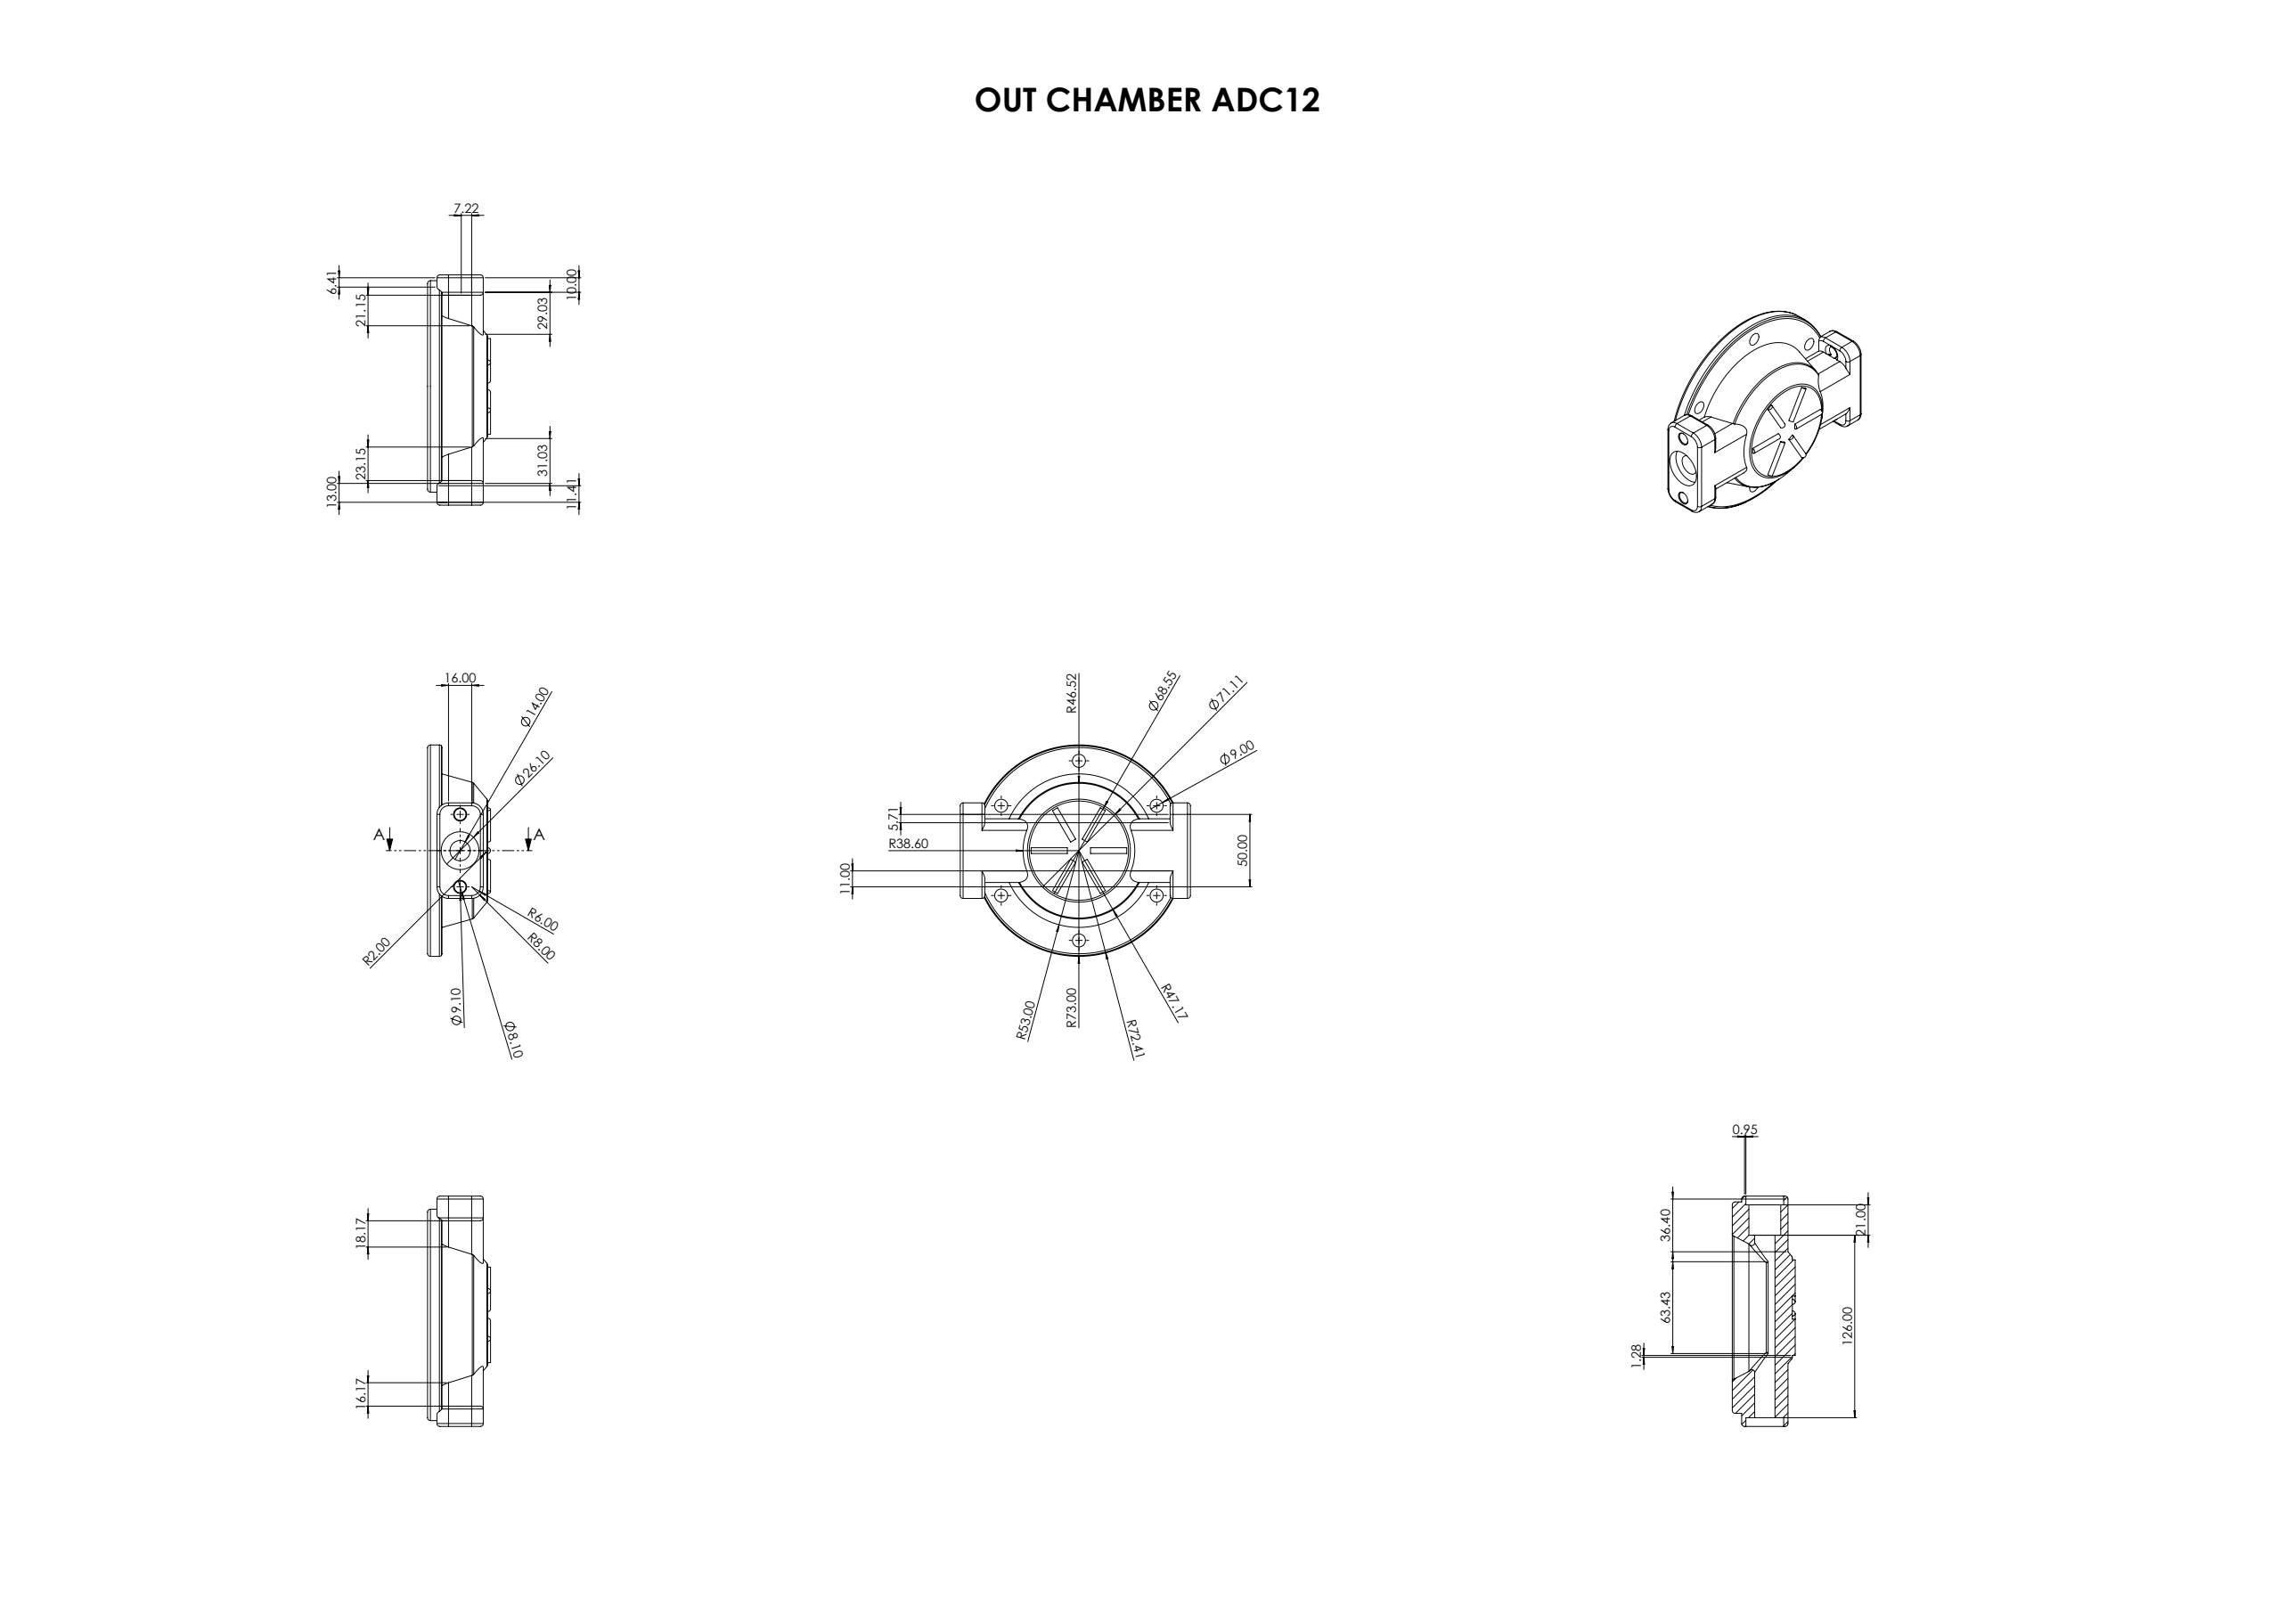
ISO-10303-21;
HEADER;
/* Generated by software containing ST-Developer
 * from STEP Tools, Inc. (www.steptools.com) 
 */

FILE_DESCRIPTION(
/* description */ (''),
/* implementation_level */ '2;1');

FILE_NAME(
/* name */ '01_Out_Chamber_ADC12.step',
/* time_stamp */ '2026-10-26T06:13:19-07:00',
/* author */ (''),
/* organization */ (''),
/* preprocessor_version */ 'ST-DEVELOPER v20.2',
/* originating_system */ 'Autodesk Translation Framework v15.15.0.0',
/* authorisation */ '');

FILE_SCHEMA (('AUTOMOTIVE_DESIGN { 1 0 10303 214 3 1 1 }','TECHNICAL_DATA_PACKAGING'));
ENDSEC;

DATA;
#10=MECHANICAL_DESIGN_GEOMETRIC_PRESENTATION_REPRESENTATION('',(#297),#56639);
#257=SHAPE_REPRESENTATION_RELATIONSHIP('SRR','None',#56745,#277);
#277=ADVANCED_BREP_SHAPE_REPRESENTATION('',(#317),#56619);
#297=STYLED_ITEM('',(#56908),#317);
#317=MANIFOLD_SOLID_BREP('Body1',#16949);
#337=B_SPLINE_SURFACE_WITH_KNOTS('',3,3,((#23722,#23723,#23724,#23725,#23726,
#23727,#23728,#23729,#23730,#23731,#23732,#23733,#23734,#23735),(#23736,
#23737,#23738,#23739,#23740,#23741,#23742,#23743,#23744,#23745,#23746,#23747,
#23748,#23749),(#23750,#23751,#23752,#23753,#23754,#23755,#23756,#23757,
#23758,#23759,#23760,#23761,#23762,#23763),(#23764,#23765,#23766,#23767,
#23768,#23769,#23770,#23771,#23772,#23773,#23774,#23775,#23776,#23777),
(#23778,#23779,#23780,#23781,#23782,#23783,#23784,#23785,#23786,#23787,
#23788,#23789,#23790,#23791),(#23792,#23793,#23794,#23795,#23796,#23797,
#23798,#23799,#23800,#23801,#23802,#23803,#23804,#23805),(#23806,#23807,
#23808,#23809,#23810,#23811,#23812,#23813,#23814,#23815,#23816,#23817,#23818,
#23819)),.UNSPECIFIED.,.F.,.F.,.F.,(4,1,1,1,4),(4,1,1,1,1,1,1,1,1,1,1,4),
(0.,0.285714285714286,0.571428571428571,0.785714285714286,1.),(4.69190485072485,
5.32399487973813,5.95608490875141,6.27212992325805,6.58817493776469,6.79887161410245,
7.00956829044021,7.22026496677797,7.43096164311573,7.85235499579125,8.48444502480452,
9.1165350538178),.UNSPECIFIED.);
#338=B_SPLINE_SURFACE_WITH_KNOTS('',3,3,((#24134,#24135,#24136,#24137,#24138,
#24139,#24140,#24141,#24142,#24143,#24144,#24145,#24146,#24147,#24148),
(#24149,#24150,#24151,#24152,#24153,#24154,#24155,#24156,#24157,#24158,
#24159,#24160,#24161,#24162,#24163),(#24164,#24165,#24166,#24167,#24168,
#24169,#24170,#24171,#24172,#24173,#24174,#24175,#24176,#24177,#24178),
(#24179,#24180,#24181,#24182,#24183,#24184,#24185,#24186,#24187,#24188,
#24189,#24190,#24191,#24192,#24193),(#24194,#24195,#24196,#24197,#24198,
#24199,#24200,#24201,#24202,#24203,#24204,#24205,#24206,#24207,#24208),
(#24209,#24210,#24211,#24212,#24213,#24214,#24215,#24216,#24217,#24218,
#24219,#24220,#24221,#24222,#24223),(#24224,#24225,#24226,#24227,#24228,
#24229,#24230,#24231,#24232,#24233,#24234,#24235,#24236,#24237,#24238)),
 .UNSPECIFIED.,.F.,.F.,.F.,(4,1,1,1,4),(4,1,1,1,1,1,1,1,1,1,1,1,4),(0.,
0.285714285714286,0.571428571428571,0.785714285714286,1.),(4.69190485072485,
5.32399487973813,5.95608490875141,6.27212992325805,6.58817493776469,6.79887161410245,
7.00956829044021,7.22026496677796,7.43096164311572,7.64165831945348,7.85235499579124,
8.48444502480452,9.1165350538178),.UNSPECIFIED.);
#367=TOROIDAL_SURFACE('',#17234,45.2410588351948,2.);
#368=TOROIDAL_SURFACE('',#17239,45.2410588351948,2.);
#369=TOROIDAL_SURFACE('',#17245,34.2759001296373,2.);
#370=TOROIDAL_SURFACE('',#17254,71.1954923578975,2.);
#371=TOROIDAL_SURFACE('',#17261,71.,2.);
#372=TOROIDAL_SURFACE('',#17269,71.1954923578975,2.);
#373=TOROIDAL_SURFACE('',#17276,71.,2.);
#374=TOROIDAL_SURFACE('',#17277,71.,2.);
#375=TOROIDAL_SURFACE('',#17288,6.,2.);
#376=TOROIDAL_SURFACE('',#17294,6.,2.);
#377=TOROIDAL_SURFACE('',#17306,6.00000000000001,2.);
#378=TOROIDAL_SURFACE('',#17311,6.,2.);
#379=TOROIDAL_SURFACE('',#17316,6.,2.);
#380=TOROIDAL_SURFACE('',#17321,6.,2.);
#381=TOROIDAL_SURFACE('',#17333,6.,2.);
#382=TOROIDAL_SURFACE('',#17335,6.00000000000001,2.);
#383=TOROIDAL_SURFACE('',#17340,51.1654934782503,2.);
#384=TOROIDAL_SURFACE('',#17354,6.,2.);
#385=TOROIDAL_SURFACE('',#17360,6.,2.);
#386=TOROIDAL_SURFACE('',#17371,6.05,2.);
#387=TOROIDAL_SURFACE('',#17373,6.00000000000001,2.);
#388=TOROIDAL_SURFACE('',#17379,6.,2.);
#389=TOROIDAL_SURFACE('',#17384,6.,2.);
#390=TOROIDAL_SURFACE('',#17388,6.,2.);
#391=TOROIDAL_SURFACE('',#17398,6.00000000000001,2.);
#392=TOROIDAL_SURFACE('',#17403,6.,2.);
#393=TOROIDAL_SURFACE('',#17412,6.05,2.);
#414=FACE_BOUND('',#2788,.T.);
#415=FACE_BOUND('',#2789,.T.);
#416=FACE_BOUND('',#2790,.T.);
#417=FACE_BOUND('',#2794,.T.);
#418=FACE_BOUND('',#2795,.T.);
#419=FACE_BOUND('',#2796,.T.);
#420=FACE_BOUND('',#2807,.T.);
#421=FACE_BOUND('',#2808,.T.);
#422=FACE_BOUND('',#2809,.T.);
#423=FACE_BOUND('',#2810,.T.);
#424=FACE_BOUND('',#2811,.T.);
#425=FACE_BOUND('',#2812,.T.);
#426=FACE_BOUND('',#2815,.T.);
#427=FACE_BOUND('',#2816,.T.);
#428=FACE_BOUND('',#2817,.T.);
#429=FACE_BOUND('',#2822,.T.);
#430=FACE_BOUND('',#2823,.T.);
#431=FACE_BOUND('',#2824,.T.);
#432=FACE_BOUND('',#2828,.T.);
#433=FACE_BOUND('',#2829,.T.);
#434=FACE_BOUND('',#2830,.T.);
#435=FACE_BOUND('',#2831,.T.);
#436=FACE_BOUND('',#2832,.T.);
#437=FACE_BOUND('',#2833,.T.);
#438=FACE_BOUND('',#2834,.T.);
#439=FACE_BOUND('',#2922,.T.);
#440=FACE_BOUND('',#2925,.T.);
#441=FACE_BOUND('',#2927,.T.);
#564=CONICAL_SURFACE('',#17208,4.3,0.785398163397448);
#565=CONICAL_SURFACE('',#17217,4.3,0.785398163397448);
#566=CONICAL_SURFACE('',#17218,4.3,0.785398163397439);
#567=CONICAL_SURFACE('',#17230,4.3,0.785398163397439);
#568=CONICAL_SURFACE('',#17237,50.,0.272145890531187);
#569=CONICAL_SURFACE('',#17243,50.,0.272145890531187);
#570=CONICAL_SURFACE('',#17250,41.,0.876058050598193);
#571=CONICAL_SURFACE('',#17344,47.,0.477345382373672);
#572=CONICAL_SURFACE('',#17465,38.,0.785398163397448);
#662=CIRCLE('',#17196,4.05);
#663=CIRCLE('',#17197,4.05);
#664=CIRCLE('',#17198,4.05);
#665=CIRCLE('',#17199,4.05);
#666=CIRCLE('',#17204,4.05);
#667=CIRCLE('',#17205,4.05);
#668=CIRCLE('',#17206,4.05);
#669=CIRCLE('',#17207,4.05);
#670=CIRCLE('',#17209,4.55);
#671=CIRCLE('',#17211,6.00000000000001);
#672=CIRCLE('',#17212,6.);
#673=CIRCLE('',#17213,6.);
#674=CIRCLE('',#17214,6.);
#675=CIRCLE('',#17215,4.55);
#676=CIRCLE('',#17216,13.05);
#677=CIRCLE('',#17219,4.55);
#678=CIRCLE('',#17220,4.05);
#679=CIRCLE('',#17222,6.00000000000001);
#680=CIRCLE('',#17223,6.);
#681=CIRCLE('',#17224,6.);
#682=CIRCLE('',#17225,6.);
#683=CIRCLE('',#17226,4.55);
#684=CIRCLE('',#17227,13.05);
#685=CIRCLE('',#17229,4.05);
#686=CIRCLE('',#17231,4.05);
#687=CIRCLE('',#17233,4.05);
#688=CIRCLE('',#17235,47.1674514378614);
#689=CIRCLE('',#17236,46.5214276345237);
#690=CIRCLE('',#17238,53.);
#691=CIRCLE('',#17240,47.1674514378614);
#692=CIRCLE('',#17241,46.5214276345237);
#693=CIRCLE('',#17242,46.5214276345237);
#694=CIRCLE('',#17244,53.);
#695=CIRCLE('',#17246,34.2759001296373);
#696=CIRCLE('',#17247,2.);
#697=CIRCLE('',#17248,35.5562689289663);
#698=CIRCLE('',#17249,35.5562689289663);
#699=CIRCLE('',#17251,38.6);
#700=CIRCLE('',#17252,38.6);
#701=CIRCLE('',#17255,72.4142135623731);
#702=CIRCLE('',#17256,71.1954923578975);
#703=CIRCLE('',#17258,4.5);
#704=CIRCLE('',#17259,4.5);
#705=CIRCLE('',#17260,4.5);
#706=CIRCLE('',#17262,73.);
#707=CIRCLE('',#17263,73.);
#708=CIRCLE('',#17265,73.);
#709=CIRCLE('',#17266,73.);
#710=CIRCLE('',#17267,73.);
#711=CIRCLE('',#17268,73.);
#712=CIRCLE('',#17270,72.4142135623731);
#713=CIRCLE('',#17271,71.1954923578975);
#714=CIRCLE('',#17273,4.5);
#715=CIRCLE('',#17274,4.5);
#716=CIRCLE('',#17275,4.5);
#717=CIRCLE('',#17278,2.);
#718=CIRCLE('',#17279,71.);
#719=CIRCLE('',#17281,4.5);
#720=CIRCLE('',#17282,4.5);
#721=CIRCLE('',#17283,4.5);
#722=CIRCLE('',#17284,4.5);
#723=CIRCLE('',#17285,4.5);
#724=CIRCLE('',#17286,4.5);
#725=CIRCLE('',#17287,51.1654934782503);
#726=CIRCLE('',#17289,6.);
#727=CIRCLE('',#17290,2.);
#728=CIRCLE('',#17291,8.);
#729=CIRCLE('',#17293,2.);
#730=CIRCLE('',#17295,2.);
#731=CIRCLE('',#17296,8.);
#732=CIRCLE('',#17297,6.);
#733=CIRCLE('',#17301,8.);
#734=CIRCLE('',#17302,8.00000000000001);
#735=CIRCLE('',#17304,2.);
#736=CIRCLE('',#17305,2.);
#737=CIRCLE('',#17307,2.);
#738=CIRCLE('',#17308,8.00000000000001);
#739=CIRCLE('',#17310,2.);
#740=CIRCLE('',#17312,2.);
#741=CIRCLE('',#17313,8.);
#742=CIRCLE('',#17315,2.);
#743=CIRCLE('',#17317,2.);
#744=CIRCLE('',#17318,8.);
#745=CIRCLE('',#17320,2.);
#746=CIRCLE('',#17322,8.);
#747=CIRCLE('',#17324,8.);
#748=CIRCLE('',#17327,8.00000000000001);
#749=CIRCLE('',#17329,2.);
#750=CIRCLE('',#17331,2.00000000000001);
#751=CIRCLE('',#17332,2.);
#752=CIRCLE('',#17334,6.);
#753=CIRCLE('',#17336,6.00000000000001);
#754=CIRCLE('',#17338,8.00000000000002);
#755=CIRCLE('',#17339,8.00000000000001);
#756=CIRCLE('',#17341,2.);
#757=CIRCLE('',#17342,49.3890581919384);
#758=CIRCLE('',#17343,49.3890581919384);
#759=CIRCLE('',#17345,44.);
#760=CIRCLE('',#17349,32.);
#761=CIRCLE('',#17350,32.);
#762=CIRCLE('',#17352,7.);
#763=CIRCLE('',#17353,7.);
#764=CIRCLE('',#17355,8.);
#765=CIRCLE('',#17356,2.);
#766=CIRCLE('',#17357,6.);
#767=CIRCLE('',#17359,2.);
#768=CIRCLE('',#17361,1.99999999999999);
#769=CIRCLE('',#17362,6.);
#770=CIRCLE('',#17363,8.);
#771=CIRCLE('',#17367,8.);
#772=CIRCLE('',#17369,6.05);
#773=CIRCLE('',#17370,8.);
#774=CIRCLE('',#17372,6.05);
#775=CIRCLE('',#17374,2.);
#776=CIRCLE('',#17375,2.);
#777=CIRCLE('',#17376,8.00000000000001);
#778=CIRCLE('',#17378,2.);
#779=CIRCLE('',#17380,2.);
#780=CIRCLE('',#17381,8.);
#781=CIRCLE('',#17383,2.);
#782=CIRCLE('',#17385,2.);
#783=CIRCLE('',#17387,2.);
#784=CIRCLE('',#17389,2.);
#785=CIRCLE('',#17390,8.);
#786=CIRCLE('',#17395,8.00000000000001);
#787=CIRCLE('',#17397,2.);
#788=CIRCLE('',#17399,2.);
#789=CIRCLE('',#17400,6.00000000000001);
#790=CIRCLE('',#17402,2.);
#791=CIRCLE('',#17404,6.);
#792=CIRCLE('',#17405,8.);
#793=CIRCLE('',#17407,8.00000000000001);
#794=CIRCLE('',#17408,6.05);
#795=CIRCLE('',#17410,6.05);
#796=CIRCLE('',#17411,8.00000000000002);
#797=CIRCLE('',#17414,2.);
#798=CIRCLE('',#17416,2.);
#799=CIRCLE('',#17418,2.);
#800=CIRCLE('',#17420,2.);
#801=CIRCLE('',#17422,2.);
#802=CIRCLE('',#17424,2.);
#803=CIRCLE('',#17426,2.);
#804=CIRCLE('',#17428,2.);
#805=CIRCLE('',#17430,2.);
#806=CIRCLE('',#17432,2.);
#807=CIRCLE('',#17434,2.);
#808=CIRCLE('',#17436,2.);
#809=CIRCLE('',#17448,8.00000000000001);
#810=CIRCLE('',#17456,13.05);
#811=CIRCLE('',#17458,11.);
#812=CIRCLE('',#17460,11.);
#813=CIRCLE('',#17463,13.05);
#814=CIRCLE('',#17466,32.);
#1226=CYLINDRICAL_SURFACE('',#17195,4.05);
#1227=CYLINDRICAL_SURFACE('',#17203,4.05);
#1228=CYLINDRICAL_SURFACE('',#17228,4.05);
#1229=CYLINDRICAL_SURFACE('',#17232,4.05);
#1230=CYLINDRICAL_SURFACE('',#17264,73.);
#1231=CYLINDRICAL_SURFACE('',#17292,2.);
#1232=CYLINDRICAL_SURFACE('',#17298,2.);
#1233=CYLINDRICAL_SURFACE('',#17303,2.);
#1234=CYLINDRICAL_SURFACE('',#17309,2.);
#1235=CYLINDRICAL_SURFACE('',#17314,2.);
#1236=CYLINDRICAL_SURFACE('',#17319,2.);
#1237=CYLINDRICAL_SURFACE('',#17323,8.);
#1238=CYLINDRICAL_SURFACE('',#17326,8.00000000000001);
#1239=CYLINDRICAL_SURFACE('',#17328,2.);
#1240=CYLINDRICAL_SURFACE('',#17330,2.);
#1241=CYLINDRICAL_SURFACE('',#17346,2.);
#1242=CYLINDRICAL_SURFACE('',#17347,2.);
#1243=CYLINDRICAL_SURFACE('',#17351,7.);
#1244=CYLINDRICAL_SURFACE('',#17358,2.);
#1245=CYLINDRICAL_SURFACE('',#17364,2.);
#1246=CYLINDRICAL_SURFACE('',#17366,8.);
#1247=CYLINDRICAL_SURFACE('',#17377,2.);
#1248=CYLINDRICAL_SURFACE('',#17382,2.);
#1249=CYLINDRICAL_SURFACE('',#17386,2.);
#1250=CYLINDRICAL_SURFACE('',#17391,2.);
#1251=CYLINDRICAL_SURFACE('',#17392,8.);
#1252=CYLINDRICAL_SURFACE('',#17394,8.00000000000001);
#1253=CYLINDRICAL_SURFACE('',#17396,2.);
#1254=CYLINDRICAL_SURFACE('',#17401,2.);
#1255=CYLINDRICAL_SURFACE('',#17415,2.);
#1256=CYLINDRICAL_SURFACE('',#17419,2.);
#1257=CYLINDRICAL_SURFACE('',#17423,2.);
#1258=CYLINDRICAL_SURFACE('',#17427,2.);
#1259=CYLINDRICAL_SURFACE('',#17431,2.);
#1260=CYLINDRICAL_SURFACE('',#17435,2.);
#1261=CYLINDRICAL_SURFACE('',#17449,4.5);
#1262=CYLINDRICAL_SURFACE('',#17450,4.5);
#1263=CYLINDRICAL_SURFACE('',#17451,4.5);
#1264=CYLINDRICAL_SURFACE('',#17452,4.5);
#1265=CYLINDRICAL_SURFACE('',#17453,4.5);
#1266=CYLINDRICAL_SURFACE('',#17454,4.5);
#1267=CYLINDRICAL_SURFACE('',#17455,13.05);
#1268=CYLINDRICAL_SURFACE('',#17459,11.);
#1269=CYLINDRICAL_SURFACE('',#17464,13.05);
#1270=CYLINDRICAL_SURFACE('',#17468,8.);
#1271=CYLINDRICAL_SURFACE('',#17470,8.);
#1272=CYLINDRICAL_SURFACE('',#17471,8.);
#1273=CYLINDRICAL_SURFACE('',#17473,8.00000000000001);
#1274=CYLINDRICAL_SURFACE('',#17476,8.);
#1275=CYLINDRICAL_SURFACE('',#17477,8.);
#1276=CYLINDRICAL_SURFACE('',#17478,8.00000000000002);
#1277=CYLINDRICAL_SURFACE('',#17479,8.00000000000001);
#1278=CYLINDRICAL_SURFACE('',#17481,8.00000000000001);
#1279=CYLINDRICAL_SURFACE('',#17483,8.00000000000002);
#1280=CYLINDRICAL_SURFACE('',#17484,8.00000000000001);
#1761=(
BOUNDED_CURVE()
B_SPLINE_CURVE(2,(#22976,#22977,#22978),.UNSPECIFIED.,.F.,.F.)
B_SPLINE_CURVE_WITH_KNOTS((3,3),(0.,1.67588266328234),.UNSPECIFIED.)
CURVE()
GEOMETRIC_REPRESENTATION_ITEM()
RATIONAL_B_SPLINE_CURVE((1.,1.00126993326289,1.))
REPRESENTATION_ITEM('')
);
#1762=(
BOUNDED_CURVE()
B_SPLINE_CURVE(2,(#23047,#23048,#23049),.UNSPECIFIED.,.F.,.F.)
B_SPLINE_CURVE_WITH_KNOTS((3,3),(0.,1.67588266328234),.UNSPECIFIED.)
CURVE()
GEOMETRIC_REPRESENTATION_ITEM()
RATIONAL_B_SPLINE_CURVE((1.,1.00126993326289,1.))
REPRESENTATION_ITEM('')
);
#1763=(
BOUNDED_CURVE()
B_SPLINE_CURVE(2,(#23196,#23197,#23198),.UNSPECIFIED.,.F.,.F.)
B_SPLINE_CURVE_WITH_KNOTS((3,3),(0.,1.67588266328234),.UNSPECIFIED.)
CURVE()
GEOMETRIC_REPRESENTATION_ITEM()
RATIONAL_B_SPLINE_CURVE((1.,1.00126993326289,1.))
REPRESENTATION_ITEM('')
);
#1764=(
BOUNDED_CURVE()
B_SPLINE_CURVE(2,(#23235,#23236,#23237),.UNSPECIFIED.,.F.,.F.)
B_SPLINE_CURVE_WITH_KNOTS((3,3),(0.,1.67588266328234),.UNSPECIFIED.)
CURVE()
GEOMETRIC_REPRESENTATION_ITEM()
RATIONAL_B_SPLINE_CURVE((1.,1.00126993326289,1.))
REPRESENTATION_ITEM('')
);
#1805=FACE_OUTER_BOUND('',#2778,.T.);
#1806=FACE_OUTER_BOUND('',#2779,.T.);
#1807=FACE_OUTER_BOUND('',#2780,.T.);
#1808=FACE_OUTER_BOUND('',#2781,.T.);
#1809=FACE_OUTER_BOUND('',#2782,.T.);
#1810=FACE_OUTER_BOUND('',#2783,.T.);
#1811=FACE_OUTER_BOUND('',#2784,.T.);
#1812=FACE_OUTER_BOUND('',#2785,.T.);
#1813=FACE_OUTER_BOUND('',#2786,.T.);
#1814=FACE_OUTER_BOUND('',#2787,.T.);
#1815=FACE_OUTER_BOUND('',#2791,.T.);
#1816=FACE_OUTER_BOUND('',#2792,.T.);
#1817=FACE_OUTER_BOUND('',#2793,.T.);
#1818=FACE_OUTER_BOUND('',#2797,.T.);
#1819=FACE_OUTER_BOUND('',#2798,.T.);
#1820=FACE_OUTER_BOUND('',#2799,.T.);
#1821=FACE_OUTER_BOUND('',#2800,.T.);
#1822=FACE_OUTER_BOUND('',#2801,.T.);
#1823=FACE_OUTER_BOUND('',#2802,.T.);
#1824=FACE_OUTER_BOUND('',#2803,.T.);
#1825=FACE_OUTER_BOUND('',#2804,.T.);
#1826=FACE_OUTER_BOUND('',#2805,.T.);
#1827=FACE_OUTER_BOUND('',#2806,.T.);
#1828=FACE_OUTER_BOUND('',#2813,.T.);
#1829=FACE_OUTER_BOUND('',#2814,.T.);
#1830=FACE_OUTER_BOUND('',#2818,.T.);
#1831=FACE_OUTER_BOUND('',#2819,.T.);
#1832=FACE_OUTER_BOUND('',#2820,.T.);
#1833=FACE_OUTER_BOUND('',#2821,.T.);
#1834=FACE_OUTER_BOUND('',#2825,.T.);
#1835=FACE_OUTER_BOUND('',#2826,.T.);
#1836=FACE_OUTER_BOUND('',#2827,.T.);
#1837=FACE_OUTER_BOUND('',#2835,.T.);
#1838=FACE_OUTER_BOUND('',#2836,.T.);
#1839=FACE_OUTER_BOUND('',#2837,.T.);
#1840=FACE_OUTER_BOUND('',#2838,.T.);
#1841=FACE_OUTER_BOUND('',#2839,.T.);
#1842=FACE_OUTER_BOUND('',#2840,.T.);
#1843=FACE_OUTER_BOUND('',#2841,.T.);
#1844=FACE_OUTER_BOUND('',#2842,.T.);
#1845=FACE_OUTER_BOUND('',#2843,.T.);
#1846=FACE_OUTER_BOUND('',#2844,.T.);
#1847=FACE_OUTER_BOUND('',#2845,.T.);
#1848=FACE_OUTER_BOUND('',#2846,.T.);
#1849=FACE_OUTER_BOUND('',#2847,.T.);
#1850=FACE_OUTER_BOUND('',#2848,.T.);
#1851=FACE_OUTER_BOUND('',#2849,.T.);
#1852=FACE_OUTER_BOUND('',#2850,.T.);
#1853=FACE_OUTER_BOUND('',#2851,.T.);
#1854=FACE_OUTER_BOUND('',#2852,.T.);
#1855=FACE_OUTER_BOUND('',#2853,.T.);
#1856=FACE_OUTER_BOUND('',#2854,.T.);
#1857=FACE_OUTER_BOUND('',#2855,.T.);
#1858=FACE_OUTER_BOUND('',#2856,.T.);
#1859=FACE_OUTER_BOUND('',#2857,.T.);
#1860=FACE_OUTER_BOUND('',#2858,.T.);
#1861=FACE_OUTER_BOUND('',#2859,.T.);
#1862=FACE_OUTER_BOUND('',#2860,.T.);
#1863=FACE_OUTER_BOUND('',#2861,.T.);
#1864=FACE_OUTER_BOUND('',#2862,.T.);
#1865=FACE_OUTER_BOUND('',#2863,.T.);
#1866=FACE_OUTER_BOUND('',#2864,.T.);
#1867=FACE_OUTER_BOUND('',#2865,.T.);
#1868=FACE_OUTER_BOUND('',#2866,.T.);
#1869=FACE_OUTER_BOUND('',#2867,.T.);
#1870=FACE_OUTER_BOUND('',#2868,.T.);
#1871=FACE_OUTER_BOUND('',#2869,.T.);
#1872=FACE_OUTER_BOUND('',#2870,.T.);
#1873=FACE_OUTER_BOUND('',#2871,.T.);
#1874=FACE_OUTER_BOUND('',#2872,.T.);
#1875=FACE_OUTER_BOUND('',#2873,.T.);
#1876=FACE_OUTER_BOUND('',#2874,.T.);
#1877=FACE_OUTER_BOUND('',#2875,.T.);
#1878=FACE_OUTER_BOUND('',#2876,.T.);
#1879=FACE_OUTER_BOUND('',#2877,.T.);
#1880=FACE_OUTER_BOUND('',#2878,.T.);
#1881=FACE_OUTER_BOUND('',#2879,.T.);
#1882=FACE_OUTER_BOUND('',#2880,.T.);
#1883=FACE_OUTER_BOUND('',#2881,.T.);
#1884=FACE_OUTER_BOUND('',#2882,.T.);
#1885=FACE_OUTER_BOUND('',#2883,.T.);
#1886=FACE_OUTER_BOUND('',#2884,.T.);
#1887=FACE_OUTER_BOUND('',#2885,.T.);
#1888=FACE_OUTER_BOUND('',#2886,.T.);
#1889=FACE_OUTER_BOUND('',#2887,.T.);
#1890=FACE_OUTER_BOUND('',#2888,.T.);
#1891=FACE_OUTER_BOUND('',#2889,.T.);
#1892=FACE_OUTER_BOUND('',#2890,.T.);
#1893=FACE_OUTER_BOUND('',#2891,.T.);
#1894=FACE_OUTER_BOUND('',#2892,.T.);
#1895=FACE_OUTER_BOUND('',#2893,.T.);
#1896=FACE_OUTER_BOUND('',#2894,.T.);
#1897=FACE_OUTER_BOUND('',#2895,.T.);
#1898=FACE_OUTER_BOUND('',#2896,.T.);
#1899=FACE_OUTER_BOUND('',#2897,.T.);
#1900=FACE_OUTER_BOUND('',#2898,.T.);
#1901=FACE_OUTER_BOUND('',#2899,.T.);
#1902=FACE_OUTER_BOUND('',#2900,.T.);
#1903=FACE_OUTER_BOUND('',#2901,.T.);
#1904=FACE_OUTER_BOUND('',#2902,.T.);
#1905=FACE_OUTER_BOUND('',#2903,.T.);
#1906=FACE_OUTER_BOUND('',#2904,.T.);
#1907=FACE_OUTER_BOUND('',#2905,.T.);
#1908=FACE_OUTER_BOUND('',#2906,.T.);
#1909=FACE_OUTER_BOUND('',#2907,.T.);
#1910=FACE_OUTER_BOUND('',#2908,.T.);
#1911=FACE_OUTER_BOUND('',#2909,.T.);
#1912=FACE_OUTER_BOUND('',#2910,.T.);
#1913=FACE_OUTER_BOUND('',#2911,.T.);
#1914=FACE_OUTER_BOUND('',#2912,.T.);
#1915=FACE_OUTER_BOUND('',#2913,.T.);
#1916=FACE_OUTER_BOUND('',#2914,.T.);
#1917=FACE_OUTER_BOUND('',#2915,.T.);
#1918=FACE_OUTER_BOUND('',#2916,.T.);
#1919=FACE_OUTER_BOUND('',#2917,.T.);
#1920=FACE_OUTER_BOUND('',#2918,.T.);
#1921=FACE_OUTER_BOUND('',#2919,.T.);
#1922=FACE_OUTER_BOUND('',#2920,.T.);
#1923=FACE_OUTER_BOUND('',#2921,.T.);
#1924=FACE_OUTER_BOUND('',#2923,.T.);
#1925=FACE_OUTER_BOUND('',#2924,.T.);
#1926=FACE_OUTER_BOUND('',#2926,.T.);
#1927=FACE_OUTER_BOUND('',#2928,.T.);
#1928=FACE_OUTER_BOUND('',#2929,.T.);
#1929=FACE_OUTER_BOUND('',#2930,.T.);
#1930=FACE_OUTER_BOUND('',#2931,.T.);
#1931=FACE_OUTER_BOUND('',#2932,.T.);
#1932=FACE_OUTER_BOUND('',#2933,.T.);
#1933=FACE_OUTER_BOUND('',#2934,.T.);
#1934=FACE_OUTER_BOUND('',#2935,.T.);
#1935=FACE_OUTER_BOUND('',#2936,.T.);
#1936=FACE_OUTER_BOUND('',#2937,.T.);
#1937=FACE_OUTER_BOUND('',#2938,.T.);
#1938=FACE_OUTER_BOUND('',#2939,.T.);
#1939=FACE_OUTER_BOUND('',#2940,.T.);
#1940=FACE_OUTER_BOUND('',#2941,.T.);
#1941=FACE_OUTER_BOUND('',#2942,.T.);
#1942=FACE_OUTER_BOUND('',#2943,.T.);
#1943=FACE_OUTER_BOUND('',#2944,.T.);
#1944=FACE_OUTER_BOUND('',#2945,.T.);
#1945=FACE_OUTER_BOUND('',#2946,.T.);
#1946=FACE_OUTER_BOUND('',#2947,.T.);
#2778=EDGE_LOOP('',(#10764,#10765,#10766,#10767));
#2779=EDGE_LOOP('',(#10768,#10769,#10770,#10771,#10772,#10773,#10774,#10775,
#10776,#10777));
#2780=EDGE_LOOP('',(#10778,#10779,#10780,#10781));
#2781=EDGE_LOOP('',(#10782,#10783,#10784,#10785,#10786,#10787,#10788,#10789));
#2782=EDGE_LOOP('',(#10790,#10791,#10792,#10793));
#2783=EDGE_LOOP('',(#10794,#10795,#10796,#10797,#10798,#10799,#10800,#10801,
#10802,#10803));
#2784=EDGE_LOOP('',(#10804,#10805,#10806,#10807));
#2785=EDGE_LOOP('',(#10808,#10809,#10810,#10811,#10812,#10813,#10814,#10815));
#2786=EDGE_LOOP('',(#10816,#10817,#10818,#10819));
#2787=EDGE_LOOP('',(#10820,#10821,#10822,#10823,#10824,#10825,#10826,#10827));
#2788=EDGE_LOOP('',(#10828));
#2789=EDGE_LOOP('',(#10829));
#2790=EDGE_LOOP('',(#10830));
#2791=EDGE_LOOP('',(#10831,#10832,#10833,#10834));
#2792=EDGE_LOOP('',(#10835,#10836,#10837,#10838));
#2793=EDGE_LOOP('',(#10839,#10840,#10841,#10842,#10843,#10844,#10845,#10846));
#2794=EDGE_LOOP('',(#10847));
#2795=EDGE_LOOP('',(#10848));
#2796=EDGE_LOOP('',(#10849));
#2797=EDGE_LOOP('',(#10850,#10851,#10852,#10853));
#2798=EDGE_LOOP('',(#10854,#10855,#10856,#10857));
#2799=EDGE_LOOP('',(#10858,#10859,#10860,#10861));
#2800=EDGE_LOOP('',(#10862,#10863,#10864,#10865));
#2801=EDGE_LOOP('',(#10866,#10867,#10868,#10869,#10870,#10871,#10872,#10873));
#2802=EDGE_LOOP('',(#10874,#10875,#10876,#10877,#10878));
#2803=EDGE_LOOP('',(#10879,#10880,#10881,#10882,#10883,#10884,#10885,#10886));
#2804=EDGE_LOOP('',(#10887,#10888,#10889,#10890,#10891));
#2805=EDGE_LOOP('',(#10892,#10893,#10894,#10895,#10896,#10897,#10898,#10899,
#10900,#10901,#10902,#10903,#10904));
#2806=EDGE_LOOP('',(#10905));
#2807=EDGE_LOOP('',(#10906,#10907,#10908,#10909));
#2808=EDGE_LOOP('',(#10910,#10911,#10912,#10913));
#2809=EDGE_LOOP('',(#10914,#10915,#10916,#10917));
#2810=EDGE_LOOP('',(#10918,#10919,#10920,#10921));
#2811=EDGE_LOOP('',(#10922,#10923,#10924,#10925));
#2812=EDGE_LOOP('',(#10926,#10927,#10928,#10929));
#2813=EDGE_LOOP('',(#10930,#10931,#10932,#10933,#10934));
#2814=EDGE_LOOP('',(#10935,#10936,#10937,#10938,#10939,#10940,#10941,#10942));
#2815=EDGE_LOOP('',(#10943));
#2816=EDGE_LOOP('',(#10944));
#2817=EDGE_LOOP('',(#10945));
#2818=EDGE_LOOP('',(#10946,#10947,#10948,#10949,#10950));
#2819=EDGE_LOOP('',(#10951,#10952,#10953,#10954,#10955,#10956,#10957,#10958,
#10959,#10960,#10961,#10962,#10963,#10964));
#2820=EDGE_LOOP('',(#10965,#10966,#10967,#10968,#10969));
#2821=EDGE_LOOP('',(#10970,#10971,#10972,#10973,#10974,#10975,#10976,#10977));
#2822=EDGE_LOOP('',(#10978));
#2823=EDGE_LOOP('',(#10979));
#2824=EDGE_LOOP('',(#10980));
#2825=EDGE_LOOP('',(#10981,#10982,#10983,#10984));
#2826=EDGE_LOOP('',(#10985,#10986,#10987,#10988));
#2827=EDGE_LOOP('',(#10989));
#2828=EDGE_LOOP('',(#10990));
#2829=EDGE_LOOP('',(#10991));
#2830=EDGE_LOOP('',(#10992));
#2831=EDGE_LOOP('',(#10993));
#2832=EDGE_LOOP('',(#10994));
#2833=EDGE_LOOP('',(#10995));
#2834=EDGE_LOOP('',(#10996));
#2835=EDGE_LOOP('',(#10997,#10998,#10999,#11000,#11001,#11002,#11003));
#2836=EDGE_LOOP('',(#11004,#11005,#11006,#11007));
#2837=EDGE_LOOP('',(#11008,#11009,#11010,#11011));
#2838=EDGE_LOOP('',(#11012,#11013,#11014,#11015));
#2839=EDGE_LOOP('',(#11016,#11017,#11018,#11019,#11020,#11021,#11022,#11023));
#2840=EDGE_LOOP('',(#11024,#11025,#11026,#11027,#11028,#11029,#11030,#11031));
#2841=EDGE_LOOP('',(#11032,#11033,#11034,#11035));
#2842=EDGE_LOOP('',(#11036,#11037,#11038,#11039));
#2843=EDGE_LOOP('',(#11040,#11041,#11042,#11043));
#2844=EDGE_LOOP('',(#11044,#11045,#11046,#11047));
#2845=EDGE_LOOP('',(#11048,#11049,#11050,#11051));
#2846=EDGE_LOOP('',(#11052,#11053,#11054,#11055));
#2847=EDGE_LOOP('',(#11056,#11057,#11058,#11059));
#2848=EDGE_LOOP('',(#11060,#11061,#11062,#11063));
#2849=EDGE_LOOP('',(#11064,#11065,#11066,#11067,#11068));
#2850=EDGE_LOOP('',(#11069,#11070,#11071,#11072));
#2851=EDGE_LOOP('',(#11073,#11074,#11075,#11076));
#2852=EDGE_LOOP('',(#11077,#11078,#11079,#11080));
#2853=EDGE_LOOP('',(#11081,#11082,#11083,#11084));
#2854=EDGE_LOOP('',(#11085,#11086,#11087,#11088,#11089,#11090,#11091));
#2855=EDGE_LOOP('',(#11092,#11093,#11094,#11095));
#2856=EDGE_LOOP('',(#11096,#11097,#11098,#11099,#11100,#11101,#11102,#11103));
#2857=EDGE_LOOP('',(#11104,#11105,#11106,#11107,#11108));
#2858=EDGE_LOOP('',(#11109,#11110,#11111,#11112,#11113));
#2859=EDGE_LOOP('',(#11114,#11115,#11116,#11117,#11118,#11119,#11120));
#2860=EDGE_LOOP('',(#11121,#11122,#11123,#11124,#11125,#11126));
#2861=EDGE_LOOP('',(#11127,#11128,#11129,#11130,#11131,#11132));
#2862=EDGE_LOOP('',(#11133,#11134,#11135,#11136,#11137,#11138,#11139));
#2863=EDGE_LOOP('',(#11140,#11141,#11142));
#2864=EDGE_LOOP('',(#11143,#11144,#11145,#11146,#11147,#11148,#11149,#11150,
#11151,#11152,#11153,#11154));
#2865=EDGE_LOOP('',(#11155,#11156,#11157,#11158,#11159));
#2866=EDGE_LOOP('',(#11160,#11161,#11162,#11163,#11164,#11165));
#2867=EDGE_LOOP('',(#11166,#11167,#11168,#11169));
#2868=EDGE_LOOP('',(#11170,#11171,#11172,#11173));
#2869=EDGE_LOOP('',(#11174,#11175,#11176,#11177));
#2870=EDGE_LOOP('',(#11178,#11179,#11180,#11181,#11182,#11183,#11184));
#2871=EDGE_LOOP('',(#11185,#11186,#11187,#11188,#11189,#11190));
#2872=EDGE_LOOP('',(#11191,#11192,#11193,#11194,#11195,#11196,#11197,#11198,
#11199));
#2873=EDGE_LOOP('',(#11200,#11201,#11202,#11203));
#2874=EDGE_LOOP('',(#11204,#11205,#11206,#11207));
#2875=EDGE_LOOP('',(#11208,#11209,#11210,#11211));
#2876=EDGE_LOOP('',(#11212,#11213,#11214,#11215));
#2877=EDGE_LOOP('',(#11216,#11217,#11218,#11219));
#2878=EDGE_LOOP('',(#11220,#11221,#11222,#11223));
#2879=EDGE_LOOP('',(#11224,#11225,#11226,#11227));
#2880=EDGE_LOOP('',(#11228,#11229,#11230,#11231));
#2881=EDGE_LOOP('',(#11232,#11233,#11234,#11235));
#2882=EDGE_LOOP('',(#11236,#11237,#11238,#11239,#11240,#11241,#11242,#11243));
#2883=EDGE_LOOP('',(#11244,#11245,#11246,#11247));
#2884=EDGE_LOOP('',(#11248,#11249,#11250,#11251));
#2885=EDGE_LOOP('',(#11252,#11253,#11254,#11255));
#2886=EDGE_LOOP('',(#11256,#11257,#11258,#11259,#11260,#11261));
#2887=EDGE_LOOP('',(#11262,#11263,#11264,#11265,#11266));
#2888=EDGE_LOOP('',(#11267,#11268,#11269,#11270,#11271,#11272));
#2889=EDGE_LOOP('',(#11273,#11274,#11275,#11276,#11277,#11278));
#2890=EDGE_LOOP('',(#11279,#11280,#11281,#11282,#11283,#11284,#11285,#11286,
#11287));
#2891=EDGE_LOOP('',(#11288,#11289));
#2892=EDGE_LOOP('',(#11290,#11291,#11292,#11293));
#2893=EDGE_LOOP('',(#11294,#11295));
#2894=EDGE_LOOP('',(#11296,#11297,#11298,#11299));
#2895=EDGE_LOOP('',(#11300,#11301));
#2896=EDGE_LOOP('',(#11302,#11303,#11304,#11305));
#2897=EDGE_LOOP('',(#11306,#11307));
#2898=EDGE_LOOP('',(#11308,#11309,#11310,#11311));
#2899=EDGE_LOOP('',(#11312,#11313));
#2900=EDGE_LOOP('',(#11314,#11315,#11316,#11317));
#2901=EDGE_LOOP('',(#11318,#11319));
#2902=EDGE_LOOP('',(#11320,#11321,#11322,#11323));
#2903=EDGE_LOOP('',(#11324,#11325));
#2904=EDGE_LOOP('',(#11326,#11327));
#2905=EDGE_LOOP('',(#11328,#11329));
#2906=EDGE_LOOP('',(#11330,#11331));
#2907=EDGE_LOOP('',(#11332,#11333));
#2908=EDGE_LOOP('',(#11334,#11335));
#2909=EDGE_LOOP('',(#11336));
#2910=EDGE_LOOP('',(#11337));
#2911=EDGE_LOOP('',(#11338,#11339,#11340,#11341));
#2912=EDGE_LOOP('',(#11342,#11343,#11344,#11345));
#2913=EDGE_LOOP('',(#11346,#11347,#11348,#11349,#11350,#11351));
#2914=EDGE_LOOP('',(#11352,#11353,#11354,#11355));
#2915=EDGE_LOOP('',(#11356,#11357,#11358,#11359));
#2916=EDGE_LOOP('',(#11360,#11361,#11362,#11363));
#2917=EDGE_LOOP('',(#11364,#11365,#11366,#11367));
#2918=EDGE_LOOP('',(#11368,#11369,#11370,#11371));
#2919=EDGE_LOOP('',(#11372,#11373,#11374,#11375));
#2920=EDGE_LOOP('',(#11376,#11377,#11378,#11379));
#2921=EDGE_LOOP('',(#11380));
#2922=EDGE_LOOP('',(#11381));
#2923=EDGE_LOOP('',(#11382,#11383,#11384,#11385));
#2924=EDGE_LOOP('',(#11386));
#2925=EDGE_LOOP('',(#11387));
#2926=EDGE_LOOP('',(#11388));
#2927=EDGE_LOOP('',(#11389));
#2928=EDGE_LOOP('',(#11390,#11391,#11392,#11393));
#2929=EDGE_LOOP('',(#11394,#11395,#11396,#11397,#11398,#11399,#11400,#11401,
#11402,#11403,#11404,#11405,#11406,#11407,#11408,#11409));
#2930=EDGE_LOOP('',(#11410,#11411));
#2931=EDGE_LOOP('',(#11412,#11413,#11414,#11415));
#2932=EDGE_LOOP('',(#11416,#11417,#11418,#11419));
#2933=EDGE_LOOP('',(#11420,#11421,#11422,#11423,#11424));
#2934=EDGE_LOOP('',(#11425,#11426,#11427,#11428,#11429,#11430,#11431));
#2935=EDGE_LOOP('',(#11432,#11433,#11434,#11435));
#2936=EDGE_LOOP('',(#11436,#11437,#11438,#11439));
#2937=EDGE_LOOP('',(#11440,#11441,#11442,#11443));
#2938=EDGE_LOOP('',(#11444,#11445,#11446,#11447));
#2939=EDGE_LOOP('',(#11448,#11449,#11450,#11451));
#2940=EDGE_LOOP('',(#11452,#11453,#11454,#11455));
#2941=EDGE_LOOP('',(#11456,#11457,#11458,#11459,#11460,#11461,#11462));
#2942=EDGE_LOOP('',(#11463,#11464,#11465,#11466,#11467,#11468,#11469));
#2943=EDGE_LOOP('',(#11470,#11471,#11472,#11473));
#2944=EDGE_LOOP('',(#11474,#11475,#11476,#11477));
#2945=EDGE_LOOP('',(#11478,#11479,#11480,#11481));
#2946=EDGE_LOOP('',(#11482,#11483,#11484,#11485,#11486,#11487,#11488));
#2947=EDGE_LOOP('',(#11489,#11490,#11491,#11492,#11493,#11494,#11495));
#3901=LINE('',#22955,#4855);
#3902=LINE('',#22957,#4856);
#3903=LINE('',#22958,#4857);
#3904=LINE('',#22961,#4858);
#3905=LINE('',#22972,#4859);
#3906=LINE('',#22974,#4860);
#3907=LINE('',#22980,#4861);
#3908=LINE('',#22982,#4862);
#3909=LINE('',#22992,#4863);
#3910=LINE('',#23004,#4864);
#3911=LINE('',#23005,#4865);
#3912=LINE('',#23010,#4866);
#3913=LINE('',#23026,#4867);
#3914=LINE('',#23028,#4868);
#3915=LINE('',#23029,#4869);
#3916=LINE('',#23032,#4870);
#3917=LINE('',#23043,#4871);
#3918=LINE('',#23045,#4872);
#3919=LINE('',#23051,#4873);
#3920=LINE('',#23053,#4874);
#3921=LINE('',#23063,#4875);
#3922=LINE('',#23075,#4876);
#3923=LINE('',#23076,#4877);
#3924=LINE('',#23081,#4878);
#3925=LINE('',#23088,#4879);
#3926=LINE('',#23094,#4880);
#3927=LINE('',#23098,#4881);
#3928=LINE('',#23102,#4882);
#3929=LINE('',#23105,#4883);
#3930=LINE('',#23111,#4884);
#3931=LINE('',#23116,#4885);
#3932=LINE('',#23121,#4886);
#3933=LINE('',#23125,#4887);
#3934=LINE('',#23129,#4888);
#3935=LINE('',#23133,#4889);
#3936=LINE('',#23141,#4890);
#3937=LINE('',#23145,#4891);
#3938=LINE('',#23149,#4892);
#3939=LINE('',#23266,#4893);
#3940=LINE('',#23334,#4894);
#3941=LINE('',#23336,#4895);
#3942=LINE('',#23338,#4896);
#3943=LINE('',#23339,#4897);
#3944=LINE('',#23342,#4898);
#3945=LINE('',#23344,#4899);
#3946=LINE('',#23346,#4900);
#3947=LINE('',#23347,#4901);
#3948=LINE('',#23350,#4902);
#3949=LINE('',#23352,#4903);
#3950=LINE('',#23354,#4904);
#3951=LINE('',#23355,#4905);
#3952=LINE('',#23358,#4906);
#3953=LINE('',#23360,#4907);
#3954=LINE('',#23362,#4908);
#3955=LINE('',#23363,#4909);
#3956=LINE('',#23366,#4910);
#3957=LINE('',#23368,#4911);
#3958=LINE('',#23370,#4912);
#3959=LINE('',#23371,#4913);
#3960=LINE('',#23374,#4914);
#3961=LINE('',#23376,#4915);
#3962=LINE('',#23378,#4916);
#3963=LINE('',#23379,#4917);
#3964=LINE('',#23423,#4918);
#3965=LINE('',#23424,#4919);
#3966=LINE('',#23426,#4920);
#3967=LINE('',#23428,#4921);
#3968=LINE('',#23504,#4922);
#3969=LINE('',#23543,#4923);
#3970=LINE('',#23544,#4924);
#3971=LINE('',#23546,#4925);
#3972=LINE('',#23548,#4926);
#3973=LINE('',#23609,#4927);
#3974=LINE('',#23610,#4928);
#3975=LINE('',#23626,#4929);
#3976=LINE('',#23627,#4930);
#3977=LINE('',#23629,#4931);
#3978=LINE('',#23631,#4932);
#3979=LINE('',#23633,#4933);
#3980=LINE('',#23635,#4934);
#3981=LINE('',#23637,#4935);
#3982=LINE('',#23638,#4936);
#3983=LINE('',#23643,#4937);
#3984=LINE('',#23655,#4938);
#3985=LINE('',#23663,#4939);
#3986=LINE('',#23671,#4940);
#3987=LINE('',#23676,#4941);
#3988=LINE('',#23678,#4942);
#3989=LINE('',#23681,#4943);
#3990=LINE('',#23682,#4944);
#3991=LINE('',#23695,#4945);
#3992=LINE('',#23700,#4946);
#3993=LINE('',#23710,#4947);
#3994=LINE('',#23720,#4948);
#3995=LINE('',#24053,#4949);
#3996=LINE('',#24060,#4950);
#3997=LINE('',#24112,#4951);
#3998=LINE('',#24118,#4952);
#3999=LINE('',#24415,#4953);
#4000=LINE('',#24417,#4954);
#4001=LINE('',#24438,#4955);
#4002=LINE('',#24440,#4956);
#4003=LINE('',#24443,#4957);
#4004=LINE('',#24459,#4958);
#4005=LINE('',#24460,#4959);
#4006=LINE('',#24463,#4960);
#4007=LINE('',#24465,#4961);
#4008=LINE('',#24466,#4962);
#4009=LINE('',#24469,#4963);
#4010=LINE('',#24485,#4964);
#4011=LINE('',#24492,#4965);
#4012=LINE('',#24502,#4966);
#4013=LINE('',#24504,#4967);
#4014=LINE('',#24507,#4968);
#4015=LINE('',#24509,#4969);
#4016=LINE('',#24510,#4970);
#4017=LINE('',#24511,#4971);
#4018=LINE('',#24514,#4972);
#4019=LINE('',#24520,#4973);
#4020=LINE('',#24544,#4974);
#4021=LINE('',#24546,#4975);
#4022=LINE('',#24549,#4976);
#4023=LINE('',#24597,#4977);
#4024=LINE('',#24599,#4978);
#4025=LINE('',#24601,#4979);
#4026=LINE('',#24603,#4980);
#4027=LINE('',#24605,#4981);
#4028=LINE('',#24607,#4982);
#4029=LINE('',#24610,#4983);
#4030=LINE('',#24617,#4984);
#4031=LINE('',#24624,#4985);
#4032=LINE('',#24626,#4986);
#4033=LINE('',#24630,#4987);
#4034=LINE('',#24632,#4988);
#4035=LINE('',#24634,#4989);
#4036=LINE('',#24636,#4990);
#4037=LINE('',#24637,#4991);
#4038=LINE('',#24644,#4992);
#4039=LINE('',#24648,#4993);
#4040=LINE('',#24650,#4994);
#4041=LINE('',#24652,#4995);
#4855=VECTOR('',#18795,10.);
#4856=VECTOR('',#18796,10.);
#4857=VECTOR('',#18797,10.);
#4858=VECTOR('',#18800,10.);
#4859=VECTOR('',#18801,10.);
#4860=VECTOR('',#18802,10.);
#4861=VECTOR('',#18803,10.);
#4862=VECTOR('',#18804,10.);
#4863=VECTOR('',#18805,10.);
#4864=VECTOR('',#18808,10.);
#4865=VECTOR('',#18809,10.);
#4866=VECTOR('',#18814,4.05);
#4867=VECTOR('',#18823,10.);
#4868=VECTOR('',#18824,10.);
#4869=VECTOR('',#18825,10.);
#4870=VECTOR('',#18828,10.);
#4871=VECTOR('',#18829,10.);
#4872=VECTOR('',#18830,10.);
#4873=VECTOR('',#18831,10.);
#4874=VECTOR('',#18832,10.);
#4875=VECTOR('',#18833,10.);
#4876=VECTOR('',#18836,10.);
#4877=VECTOR('',#18837,10.);
#4878=VECTOR('',#18842,4.05);
#4879=VECTOR('',#18853,4.3);
#4880=VECTOR('',#18858,10.);
#4881=VECTOR('',#18861,10.);
#4882=VECTOR('',#18864,10.);
#4883=VECTOR('',#18867,10.);
#4884=VECTOR('',#18874,4.3);
#4885=VECTOR('',#18879,4.3);
#4886=VECTOR('',#18884,10.);
#4887=VECTOR('',#18887,10.);
#4888=VECTOR('',#18890,10.);
#4889=VECTOR('',#18893,10.);
#4890=VECTOR('',#18902,4.05);
#4891=VECTOR('',#18907,4.3);
#4892=VECTOR('',#18912,4.05);
#4893=VECTOR('',#18949,41.);
#4894=VECTOR('',#18956,10.);
#4895=VECTOR('',#18957,10.);
#4896=VECTOR('',#18958,10.);
#4897=VECTOR('',#18959,10.);
#4898=VECTOR('',#18960,10.);
#4899=VECTOR('',#18961,10.);
#4900=VECTOR('',#18962,10.);
#4901=VECTOR('',#18963,10.);
#4902=VECTOR('',#18964,10.);
#4903=VECTOR('',#18965,10.);
#4904=VECTOR('',#18966,10.);
#4905=VECTOR('',#18967,10.);
#4906=VECTOR('',#18968,10.);
#4907=VECTOR('',#18969,10.);
#4908=VECTOR('',#18970,10.);
#4909=VECTOR('',#18971,10.);
#4910=VECTOR('',#18972,10.);
#4911=VECTOR('',#18973,10.);
#4912=VECTOR('',#18974,10.);
#4913=VECTOR('',#18975,10.);
#4914=VECTOR('',#18976,10.);
#4915=VECTOR('',#18977,10.);
#4916=VECTOR('',#18978,10.);
#4917=VECTOR('',#18979,10.);
#4918=VECTOR('',#18988,10.);
#4919=VECTOR('',#18989,10.);
#4920=VECTOR('',#18990,10.);
#4921=VECTOR('',#18991,10.);
#4922=VECTOR('',#19012,73.);
#4923=VECTOR('',#19023,10.);
#4924=VECTOR('',#19024,10.);
#4925=VECTOR('',#19025,10.);
#4926=VECTOR('',#19026,10.);
#4927=VECTOR('',#19069,10.);
#4928=VECTOR('',#19070,10.);
#4929=VECTOR('',#19081,10.);
#4930=VECTOR('',#19082,10.);
#4931=VECTOR('',#19085,10.);
#4932=VECTOR('',#19086,10.);
#4933=VECTOR('',#19087,10.);
#4934=VECTOR('',#19088,10.);
#4935=VECTOR('',#19089,10.);
#4936=VECTOR('',#19090,10.);
#4937=VECTOR('',#19095,10.);
#4938=VECTOR('',#19114,10.);
#4939=VECTOR('',#19125,10.);
#4940=VECTOR('',#19136,10.);
#4941=VECTOR('',#19143,10.);
#4942=VECTOR('',#19146,10.);
#4943=VECTOR('',#19149,10.);
#4944=VECTOR('',#19150,10.);
#4945=VECTOR('',#19159,10.);
#4946=VECTOR('',#19164,10.);
#4947=VECTOR('',#19179,10.);
#4948=VECTOR('',#19192,47.);
#4949=VECTOR('',#19197,10.);
#4950=VECTOR('',#19198,10.);
#4951=VECTOR('',#19201,10.);
#4952=VECTOR('',#19202,10.);
#4953=VECTOR('',#19213,7.);
#4954=VECTOR('',#19214,7.);
#4955=VECTOR('',#19227,10.);
#4956=VECTOR('',#19228,10.);
#4957=VECTOR('',#19231,10.);
#4958=VECTOR('',#19242,10.);
#4959=VECTOR('',#19243,10.);
#4960=VECTOR('',#19246,10.);
#4961=VECTOR('',#19247,10.);
#4962=VECTOR('',#19248,10.);
#4963=VECTOR('',#19251,10.);
#4964=VECTOR('',#19276,10.);
#4965=VECTOR('',#19287,10.);
#4966=VECTOR('',#19304,10.);
#4967=VECTOR('',#19307,10.);
#4968=VECTOR('',#19310,10.);
#4969=VECTOR('',#19311,10.);
#4970=VECTOR('',#19312,10.);
#4971=VECTOR('',#19313,10.);
#4972=VECTOR('',#19316,10.);
#4973=VECTOR('',#19323,10.);
#4974=VECTOR('',#19332,10.);
#4975=VECTOR('',#19333,10.);
#4976=VECTOR('',#19336,10.);
#4977=VECTOR('',#19431,4.5);
#4978=VECTOR('',#19434,4.5);
#4979=VECTOR('',#19437,4.5);
#4980=VECTOR('',#19440,4.5);
#4981=VECTOR('',#19443,4.5);
#4982=VECTOR('',#19446,4.5);
#4983=VECTOR('',#19449,13.05);
#4984=VECTOR('',#19458,11.);
#4985=VECTOR('',#19469,13.05);
#4986=VECTOR('',#19472,38.);
#4987=VECTOR('',#19479,10.);
#4988=VECTOR('',#19482,10.);
#4989=VECTOR('',#19485,10.);
#4990=VECTOR('',#19488,10.);
#4991=VECTOR('',#19489,10.);
#4992=VECTOR('',#19502,10.);
#4993=VECTOR('',#19509,10.);
#4994=VECTOR('',#19512,10.);
#4995=VECTOR('',#19515,10.);
#5809=B_SPLINE_CURVE_WITH_KNOTS('',3,(#22946,#22947,#22948,#22949,#22950,
#22951,#22952,#22953),.UNSPECIFIED.,.F.,.F.,(4,2,2,4),(0.589540352546839,
0.67637836992065,0.709007118931895,0.73245734358678),.UNSPECIFIED.);
#5810=B_SPLINE_CURVE_WITH_KNOTS('',3,(#22963,#22964,#22965,#22966,#22967,
#22968,#22969,#22970),.UNSPECIFIED.,.F.,.F.,(4,2,2,4),(0.766228943549322,
0.796165087029866,0.888720170530452,0.980335690408468),.UNSPECIFIED.);
#5811=B_SPLINE_CURVE_WITH_KNOTS('',3,(#22984,#22985,#22986,#22987,#22988,
#22989,#22990,#22991),.UNSPECIFIED.,.F.,.F.,(4,2,2,4),(0.313128211350458,
0.404743731228475,0.49729881472906,0.527234958209604),.UNSPECIFIED.);
#5812=B_SPLINE_CURVE_WITH_KNOTS('',3,(#22995,#22996,#22997,#22998,#22999,
#23000,#23001,#23002),.UNSPECIFIED.,.F.,.F.,(4,2,2,4),(0.732457343586781,
0.755907568241666,0.788536317252911,0.875374334626722),.UNSPECIFIED.);
#5813=B_SPLINE_CURVE_WITH_KNOTS('',3,(#23017,#23018,#23019,#23020,#23021,
#23022,#23023,#23024),.UNSPECIFIED.,.F.,.F.,(4,2,2,4),(0.589540352546839,
0.67637836992065,0.709007118931895,0.73245734358678),.UNSPECIFIED.);
#5814=B_SPLINE_CURVE_WITH_KNOTS('',3,(#23034,#23035,#23036,#23037,#23038,
#23039,#23040,#23041),.UNSPECIFIED.,.F.,.F.,(4,2,2,4),(0.766228943549322,
0.796165087029866,0.888720170530452,0.980335690408468),.UNSPECIFIED.);
#5815=B_SPLINE_CURVE_WITH_KNOTS('',3,(#23055,#23056,#23057,#23058,#23059,
#23060,#23061,#23062),.UNSPECIFIED.,.F.,.F.,(4,2,2,4),(0.313128211350458,
0.404743731228475,0.49729881472906,0.527234958209605),.UNSPECIFIED.);
#5816=B_SPLINE_CURVE_WITH_KNOTS('',3,(#23066,#23067,#23068,#23069,#23070,
#23071,#23072,#23073),.UNSPECIFIED.,.F.,.F.,(4,2,2,4),(0.732457343586781,
0.755907568241666,0.788536317252911,0.875374334626722),.UNSPECIFIED.);
#5817=B_SPLINE_CURVE_WITH_KNOTS('',3,(#23154,#23155,#23156,#23157,#23158,
#23159,#23160,#23161),.UNSPECIFIED.,.F.,.F.,(4,2,2,4),(0.0547106625868535,
0.0760286813703655,0.152661638492553,0.177931278217517),.UNSPECIFIED.);
#5818=B_SPLINE_CURVE_WITH_KNOTS('',3,(#23165,#23166,#23167,#23168,#23169,
#23170,#23171,#23172),.UNSPECIFIED.,.F.,.F.,(4,2,2,4),(1.17732071475277,
1.23123357712069,1.29332668906214,1.30059629306183),.UNSPECIFIED.);
#5819=B_SPLINE_CURVE_WITH_KNOTS('',3,(#23175,#23176,#23177,#23178),
 .UNSPECIFIED.,.F.,.F.,(4,4),(2.48707902657156,2.52790949335551),
 .UNSPECIFIED.);
#5820=B_SPLINE_CURVE_WITH_KNOTS('',3,(#23180,#23181,#23182,#23183,#23184,
#23185),.UNSPECIFIED.,.F.,.F.,(4,2,4),(2.51549718449135,2.75342616579224,
3.00837168949227),.UNSPECIFIED.);
#5821=B_SPLINE_CURVE_WITH_KNOTS('',3,(#23189,#23190,#23191,#23192,#23193,
#23194),.UNSPECIFIED.,.F.,.F.,(4,2,4),(2.01718694432165,2.27213246802168,
2.51006144932256),.UNSPECIFIED.);
#5822=B_SPLINE_CURVE_WITH_KNOTS('',3,(#23199,#23200,#23201,#23202),
 .UNSPECIFIED.,.F.,.F.,(4,4),(2.52245632487896,2.56328703668614),
 .UNSPECIFIED.);
#5823=B_SPLINE_CURVE_WITH_KNOTS('',3,(#23206,#23207,#23208,#23209,#23210,
#23211,#23212,#23213),.UNSPECIFIED.,.F.,.F.,(4,2,2,4),(0.0547106625868542,
0.0760286813703704,0.152661638492567,0.177931278217529),.UNSPECIFIED.);
#5824=B_SPLINE_CURVE_WITH_KNOTS('',3,(#23217,#23218,#23219,#23220,#23221,
#23222,#23223,#23224),.UNSPECIFIED.,.F.,.F.,(4,2,2,4),(1.17732071475281,
1.23123357712072,1.29332668906218,1.30059629306187),.UNSPECIFIED.);
#5825=B_SPLINE_CURVE_WITH_KNOTS('',3,(#23230,#23231,#23232,#23233),
 .UNSPECIFIED.,.F.,.F.,(4,4),(0.0652178919951661,0.106048358779118),
 .UNSPECIFIED.);
#5826=B_SPLINE_CURVE_WITH_KNOTS('',3,(#23239,#23240,#23241,#23242,#23243,
#23244),.UNSPECIFIED.,.F.,.F.,(4,2,4),(0.0969458522659179,0.334874833566804,
0.589820357266834),.UNSPECIFIED.);
#5827=B_SPLINE_CURVE_WITH_KNOTS('',3,(#23247,#23248,#23249,#23250,#23251,
#23252),.UNSPECIFIED.,.F.,.F.,(4,2,4),(4.43573827654708,4.69068380024711,
4.92861278154799),.UNSPECIFIED.);
#5828=B_SPLINE_CURVE_WITH_KNOTS('',3,(#23253,#23254,#23255,#23256),
 .UNSPECIFIED.,.F.,.F.,(4,4),(4.94431745945535,4.98514817126253),
 .UNSPECIFIED.);
#5829=B_SPLINE_CURVE_WITH_KNOTS('',3,(#23268,#23269,#23270,#23271,#23272,
#23273,#23274,#23275,#23276,#23277,#23278,#23279,#23280,#23281,#23282),
 .UNSPECIFIED.,.F.,.F.,(4,3,2,2,2,2,4),(-0.398983050648409,0.,0.303890790649899,
0.455836185974848,0.607781581299797,0.752378251432681,0.891363616487534),
 .UNSPECIFIED.);
#5830=B_SPLINE_CURVE_WITH_KNOTS('',3,(#23285,#23286,#23287,#23288,#23289,
#23290,#23291,#23292,#23293,#23294,#23295,#23296,#23297,#23298),
 .UNSPECIFIED.,.F.,.F.,(4,2,2,2,2,2,4),(1.88180040661422,2.02078577166908,
2.16538244180196,2.31732783712691,2.46927323245186,2.77316402310176,3.17214707374984),
 .UNSPECIFIED.);
#5831=B_SPLINE_CURVE_WITH_KNOTS('',3,(#23300,#23301,#23302,#23303,#23304,
#23305,#23306,#23307,#23308,#23309,#23310,#23311,#23312,#23313),
 .UNSPECIFIED.,.F.,.F.,(4,2,2,2,2,2,4),(3.33378803122811,3.7327710818762,
4.0366618725261,4.18860726785105,4.34055266317599,4.48514933330888,4.62413469836373),
 .UNSPECIFIED.);
#5832=B_SPLINE_CURVE_WITH_KNOTS('',3,(#23316,#23317,#23318,#23319,#23320,
#23321,#23322,#23323,#23324,#23325,#23326,#23327,#23328,#23329,#23330),
 .UNSPECIFIED.,.F.,.F.,(4,2,2,2,2,3,4),(-0.891363616497897,-0.752378251432681,
-0.607781581299798,-0.455836185974849,-0.303890790649899,0.,0.398983050648084),
 .UNSPECIFIED.);
#5833=B_SPLINE_CURVE_WITH_KNOTS('',3,(#23383,#23384,#23385,#23386,#23387,
#23388,#23389,#23390,#23391,#23392),.UNSPECIFIED.,.F.,.F.,(4,2,2,2,4),(-0.262282482196273,
-0.227243259123267,-0.192394209601782,-0.119607601361313,-4.76311912134264E-9),
 .UNSPECIFIED.);
#5834=B_SPLINE_CURVE_WITH_KNOTS('',3,(#23396,#23397,#23398,#23399),
 .UNSPECIFIED.,.F.,.F.,(4,4),(0.126241397614949,0.16067610951008),
 .UNSPECIFIED.);
#5835=B_SPLINE_CURVE_WITH_KNOTS('',3,(#23401,#23402,#23403,#23404,#23405,
#23406,#23407,#23408,#23409,#23410),.UNSPECIFIED.,.F.,.F.,(4,2,2,2,4),(-0.170608922894474,
-0.144436965084543,-0.118924812328332,-0.0673862936043148,-0.0387732480152514),
 .UNSPECIFIED.);
#5836=B_SPLINE_CURVE_WITH_KNOTS('',3,(#23414,#23415,#23416,#23417,#23418,
#23419,#23420,#23421),.UNSPECIFIED.,.F.,.F.,(4,2,2,4),(0.833662394778907,
0.872087702776309,0.960661189189834,1.07674525757504),.UNSPECIFIED.);
#5837=B_SPLINE_CURVE_WITH_KNOTS('',3,(#23429,#23430,#23431,#23432),
 .UNSPECIFIED.,.F.,.F.,(4,4),(0.380499979702294,0.388208254648859),
 .UNSPECIFIED.);
#5838=B_SPLINE_CURVE_WITH_KNOTS('',3,(#23441,#23442,#23443,#23444,#23445,
#23446,#23447,#23448),.UNSPECIFIED.,.F.,.F.,(4,2,2,4),(2.91893463596102,
3.23522229935707,3.48529709981458,3.66035951911029),.UNSPECIFIED.);
#5839=B_SPLINE_CURVE_WITH_KNOTS('',3,(#23453,#23454,#23455,#23456,#23457,
#23458),.UNSPECIFIED.,.F.,.F.,(4,2,4),(2.69869497051652,2.83559328791136,
2.94278637796835),.UNSPECIFIED.);
#5840=B_SPLINE_CURVE_WITH_KNOTS('',3,(#23461,#23462,#23463,#23464),
 .UNSPECIFIED.,.F.,.F.,(4,4),(1.017709791401,1.13054679723933),
 .UNSPECIFIED.);
#5841=B_SPLINE_CURVE_WITH_KNOTS('',3,(#23466,#23467,#23468,#23469,#23470,
#23471),.UNSPECIFIED.,.F.,.F.,(4,2,4),(0.833062331394999,0.930697160636575,
1.25845097237232),.UNSPECIFIED.);
#5842=B_SPLINE_CURVE_WITH_KNOTS('',3,(#23475,#23476,#23477,#23478,#23479,
#23480),.UNSPECIFIED.,.F.,.F.,(4,2,4),(1.23426399221579,1.56201780395154,
1.65965263319311),.UNSPECIFIED.);
#5843=B_SPLINE_CURVE_WITH_KNOTS('',3,(#23482,#23483,#23484,#23485),
 .UNSPECIFIED.,.F.,.F.,(4,4),(3.27413741533483,3.47407808778078),
 .UNSPECIFIED.);
#5844=B_SPLINE_CURVE_WITH_KNOTS('',3,(#23489,#23490,#23491,#23492,#23493,
#23494),.UNSPECIFIED.,.F.,.F.,(4,2,4),(3.21456009570699,3.42341212522469,
3.75116593696043),.UNSPECIFIED.);
#5845=B_SPLINE_CURVE_WITH_KNOTS('',3,(#23497,#23498,#23499,#23500,#23501,
#23502),.UNSPECIFIED.,.F.,.F.,(4,2,4),(3.72697895680391,4.05473276853965,
4.26358479805735),.UNSPECIFIED.);
#5846=B_SPLINE_CURVE_WITH_KNOTS('',3,(#23509,#23510,#23511,#23512),
 .UNSPECIFIED.,.F.,.F.,(4,4),(0.,0.034672276467981),.UNSPECIFIED.);
#5847=B_SPLINE_CURVE_WITH_KNOTS('',3,(#23516,#23517,#23518,#23519,#23520,
#23521,#23522,#23523,#23524,#23525),.UNSPECIFIED.,.F.,.F.,(4,2,2,2,4),(-0.183241852105191,
-0.122572168940508,-0.0730310763026209,-0.0347695149370618,0.),
 .UNSPECIFIED.);
#5848=B_SPLINE_CURVE_WITH_KNOTS('',3,(#23528,#23529,#23530,#23531,#23532,
#23533,#23534,#23535),.UNSPECIFIED.,.F.,.F.,(4,2,2,4),(-0.113889377457268,
-0.0824728782510042,-0.0390501696847016,0.),.UNSPECIFIED.);
#5849=B_SPLINE_CURVE_WITH_KNOTS('',3,(#23538,#23539,#23540,#23541),
 .UNSPECIFIED.,.F.,.F.,(4,4),(2.52634703651881,2.53405531146538),
 .UNSPECIFIED.);
#5850=B_SPLINE_CURVE_WITH_KNOTS('',3,(#23549,#23550,#23551,#23552,#23553,
#23554,#23555,#23556),.UNSPECIFIED.,.F.,.F.,(4,2,2,4),(-1.07674525757504,
-0.960661189189834,-0.872087702776309,-0.833662394778906),.UNSPECIFIED.);
#5851=B_SPLINE_CURVE_WITH_KNOTS('',3,(#23564,#23565,#23566,#23567,#23568,
#23569,#23570,#23571,#23572,#23573),.UNSPECIFIED.,.F.,.F.,(4,2,2,2,4),(1.11476433242992,
1.1444058833459,1.18561459615229,1.2451591319351,1.2623152396797),
 .UNSPECIFIED.);
#5852=B_SPLINE_CURVE_WITH_KNOTS('',3,(#23574,#23575,#23576,#23577,#23578,
#23579),.UNSPECIFIED.,.F.,.F.,(4,2,4),(0.903765698424978,1.01257762815112,
1.10763430905713),.UNSPECIFIED.);
#5853=B_SPLINE_CURVE_WITH_KNOTS('',3,(#23620,#23621,#23622,#23623,#23624,
#23625),.UNSPECIFIED.,.F.,.F.,(4,2,4),(0.,0.299277276892222,0.598554553784445),
 .UNSPECIFIED.);
#5854=B_SPLINE_CURVE_WITH_KNOTS('',3,(#23689,#23690,#23691,#23692,#23693,
#23694),.UNSPECIFIED.,.F.,.F.,(4,2,4),(1.30156425141724,1.60084152830946,
1.90011880520168),.UNSPECIFIED.);
#5855=B_SPLINE_CURVE_WITH_KNOTS('',3,(#23822,#23823,#23824,#23825,#23826,
#23827,#23828,#23829,#23830,#23831,#23832,#23833,#23834,#23835,#23836,#23837,
#23838,#23839,#23840,#23841,#23842,#23843,#23844,#23845,#23846,#23847,#23848,
#23849,#23850,#23851,#23852,#23853,#23854,#23855,#23856,#23857,#23858,#23859,
#23860,#23861,#23862,#23863,#23864,#23865,#23866,#23867,#23868,#23869,#23870,
#23871,#23872,#23873,#23874,#23875,#23876,#23877,#23878,#23879,#23880,#23881,
#23882,#23883,#23884,#23885,#23886,#23887,#23888,#23889,#23890,#23891,#23892,
#23893,#23894,#23895,#23896,#23897,#23898,#23899,#23900,#23901,#23902,#23903,
#23904,#23905,#23906,#23907,#23908,#23909,#23910,#23911,#23912,#23913,#23914,
#23915,#23916,#23917,#23918,#23919,#23920,#23921,#23922,#23923,#23924,#23925,
#23926,#23927,#23928,#23929,#23930,#23931,#23932,#23933,#23934,#23935,#23936,
#23937,#23938,#23939,#23940,#23941,#23942,#23943,#23944,#23945,#23946,#23947,
#23948,#23949,#23950,#23951,#23952,#23953,#23954,#23955,#23956,#23957,#23958,
#23959,#23960,#23961,#23962,#23963,#23964,#23965,#23966),.UNSPECIFIED.,
 .F.,.F.,(4,3,3,3,3,3,3,3,3,3,3,3,3,3,3,3,3,3,3,3,3,3,3,3,3,3,3,3,3,3,3,
3,3,3,3,3,3,3,3,3,3,3,3,3,3,3,3,3,4),(-9.03360503529916,-8.86127604911423,
-8.68030493926038,-8.58511998488549,-8.48447670513606,-8.33562131806494,
-8.19092008514545,-8.0572821722663,-7.97401584150341,-7.8693192178446,-7.85250838613552,
-7.7529816299934,-7.65895403017618,-7.57088295203555,-7.56492643035897,
-7.43104909192891,-7.27359031327789,-7.22029805007692,-7.19153158116352,
-7.1005636564517,-7.05507969409579,-7.03145147969554,-7.01779966872338,
-7.00959573173988,-6.9345284310504,-6.9042290999944,-6.82350845623894,-6.798847127526,
-6.79827768985696,-6.73152769721655,-6.66072565278933,-6.6295195877408,
-6.58805343095027,-6.51251273433006,-6.43306219328815,-6.34686858849436,
-6.30164584299914,-6.27213715467711,-6.08350153753309,-5.95594925749777,
-5.86905659224252,-5.70894094483269,-5.53318477689864,-5.33956788736791,
-5.32383027162032,-5.15411754086443,-5.01473160504778,-4.88034698710192,
-4.77483276840798),.UNSPECIFIED.);
#5856=B_SPLINE_CURVE_WITH_KNOTS('',3,(#23968,#23969,#23970,#23971),
 .UNSPECIFIED.,.F.,.F.,(4,4),(-4.77483276840798,-4.77362713684779),
 .UNSPECIFIED.);
#5857=B_SPLINE_CURVE_WITH_KNOTS('',3,(#23973,#23974,#23975,#23976,#23977,
#23978,#23979,#23980,#23981,#23982),.UNSPECIFIED.,.F.,.F.,(4,2,2,2,4),(-0.242938279070336,
-0.168006152846838,-0.0865010676432649,0.,0.000616246384910699),
 .UNSPECIFIED.);
#5858=B_SPLINE_CURVE_WITH_KNOTS('',3,(#23984,#23985,#23986,#23987,#23988,
#23989,#23990,#23991,#23992),.UNSPECIFIED.,.F.,.F.,(4,1,1,1,1,1,4),(4.69190485072485,
5.32399487973813,5.95608490875141,6.27212992325805,6.58817493776469,6.79887161410245,
6.9042290999944),.UNSPECIFIED.);
#5859=B_SPLINE_CURVE_WITH_KNOTS('',3,(#23994,#23995,#23996,#23997,#23998,
#23999,#24000,#24001,#24002),.UNSPECIFIED.,.F.,.F.,(4,1,1,1,1,1,4),(6.90422173516042,
7.00956829044021,7.22026496677797,7.43096164311573,7.85235499579125,8.48444502480452,
9.1165350538178),.UNSPECIFIED.);
#5860=B_SPLINE_CURVE_WITH_KNOTS('',3,(#24004,#24005,#24006,#24007,#24008,
#24009,#24010,#24011,#24012,#24013,#24014,#24015,#24016,#24017,#24018,#24019,
#24020,#24021,#24022,#24023,#24024,#24025,#24026,#24027,#24028,#24029,#24030,
#24031,#24032,#24033,#24034,#24035,#24036,#24037,#24038,#24039,#24040,#24041,
#24042,#24043,#24044,#24045,#24046),.UNSPECIFIED.,.F.,.F.,(4,3,3,3,3,3,
3,3,3,3,3,3,3,3,4),(-0.242801352910212,-0.242186632434824,-0.219544055688108,
-0.196801089607309,-0.174161287740677,-0.167361569498752,-0.144942724018392,
-0.122816117509345,-0.104446209841387,-0.0913857413699424,-0.0692335334813781,
-0.0520648532547955,-0.0303649913441254,-0.0155217575353379,0.),
 .UNSPECIFIED.);
#5861=B_SPLINE_CURVE_WITH_KNOTS('',3,(#24047,#24048,#24049,#24050),
 .UNSPECIFIED.,.F.,.F.,(4,4),(-9.03481070423354,-9.03360503529916),
 .UNSPECIFIED.);
#5862=B_SPLINE_CURVE_WITH_KNOTS('',3,(#24055,#24056,#24057,#24058),
 .UNSPECIFIED.,.F.,.F.,(4,4),(-1.22314360071756,-1.20515902132338),
 .UNSPECIFIED.);
#5863=B_SPLINE_CURVE_WITH_KNOTS('',3,(#24062,#24063,#24064,#24065),
 .UNSPECIFIED.,.F.,.F.,(4,4),(-0.29725330048063,-0.279268721057567),
 .UNSPECIFIED.);
#5864=B_SPLINE_CURVE_WITH_KNOTS('',3,(#24066,#24067,#24068,#24069,#24070,
#24071,#24072,#24073,#24074,#24075,#24076,#24077,#24078,#24079,#24080,#24081,
#24082,#24083,#24084,#24085,#24086,#24087,#24088,#24089,#24090,#24091,#24092,
#24093,#24094,#24095,#24096,#24097,#24098,#24099,#24100,#24101,#24102,#24103,
#24104,#24105,#24106,#24107,#24108),.UNSPECIFIED.,.F.,.F.,(4,3,3,3,3,3,
3,3,3,3,3,3,3,3,4),(-0.242801352899586,-0.242186632423413,-0.219537690406595,
-0.196781321893934,-0.174161287742756,-0.167361569500369,-0.144934602663136,
-0.12280231801636,-0.104446209842394,-0.0913857413708117,-0.0692313418368474,
-0.0520648532552464,-0.0303594951871729,-0.0155217575353938,0.),
 .UNSPECIFIED.);
#5865=B_SPLINE_CURVE_WITH_KNOTS('',3,(#24113,#24114,#24115,#24116),
 .UNSPECIFIED.,.F.,.F.,(4,4),(-0.29725330048063,-0.279268721057567),
 .UNSPECIFIED.);
#5866=B_SPLINE_CURVE_WITH_KNOTS('',3,(#24120,#24121,#24122,#24123,#24124,
#24125,#24126,#24127,#24128,#24129),.UNSPECIFIED.,.F.,.F.,(4,2,2,2,4),(-0.000616246385038109,
0.,0.0865010676321112,0.168006152835906,0.242938281746869),
 .UNSPECIFIED.);
#5867=B_SPLINE_CURVE_WITH_KNOTS('',3,(#24130,#24131,#24132,#24133),
 .UNSPECIFIED.,.F.,.F.,(4,4),(-1.22314360071756,-1.20515902132338),
 .UNSPECIFIED.);
#5868=B_SPLINE_CURVE_WITH_KNOTS('',3,(#24241,#24242,#24243,#24244,#24245,
#24246,#24247,#24248,#24249,#24250,#24251,#24252,#24253,#24254,#24255,#24256,
#24257,#24258,#24259,#24260,#24261,#24262,#24263,#24264,#24265,#24266,#24267,
#24268,#24269,#24270,#24271,#24272,#24273,#24274,#24275,#24276,#24277,#24278,
#24279,#24280,#24281,#24282,#24283,#24284,#24285,#24286,#24287,#24288,#24289,
#24290,#24291,#24292,#24293,#24294,#24295,#24296,#24297,#24298,#24299,#24300,
#24301,#24302,#24303,#24304,#24305,#24306,#24307,#24308,#24309,#24310,#24311,
#24312,#24313,#24314,#24315,#24316,#24317,#24318,#24319,#24320,#24321,#24322,
#24323,#24324,#24325,#24326,#24327,#24328,#24329,#24330,#24331,#24332,#24333,
#24334,#24335,#24336,#24337,#24338,#24339,#24340,#24341,#24342,#24343,#24344,
#24345,#24346,#24347,#24348,#24349,#24350,#24351,#24352,#24353,#24354,#24355,
#24356,#24357,#24358,#24359,#24360,#24361,#24362,#24363,#24364,#24365,#24366,
#24367,#24368,#24369,#24370,#24371,#24372,#24373,#24374,#24375,#24376,#24377,
#24378,#24379),.UNSPECIFIED.,.F.,.F.,(4,3,3,3,3,3,3,3,3,3,3,3,3,3,3,3,3,
3,3,3,3,3,3,3,3,3,3,3,3,3,3,3,3,3,3,3,3,3,3,3,3,3,3,3,3,3,4),(-9.03360503529916,
-8.88762712989133,-8.73438537212543,-8.58511998488547,-8.48471177745109,
-8.31820898189202,-8.16176952472331,-8.02347743465504,-7.97401584150339,
-7.85242356738565,-7.7130263178265,-7.64168550640925,-7.56492643035895,
-7.44264973091217,-7.43099479970612,-7.32266350526435,-7.22031662758344,
-7.20899476726769,-7.12730880556465,-7.05066524148345,-7.02706994696297,
-7.00959174062256,-6.92909838503205,-6.9042290999944,-6.8364308822668,-6.79885763435364,
-6.79827768985695,-6.73134713296141,-6.66020538781699,-6.62951958774078,
-6.58806194215221,-6.51258041717339,-6.43313965917345,-6.34691295539751,
-6.30164584299912,-6.27214200893841,-6.08189682874827,-5.95595235925663,
-5.8690565922425,-5.70909971098082,-5.53356025052748,-5.34017121243578,
-5.3238295138681,-5.1541175408644,-5.01464175348577,-4.88022674714609,-4.77483276840798),
 .UNSPECIFIED.);
#5869=B_SPLINE_CURVE_WITH_KNOTS('',3,(#24380,#24381,#24382,#24383),
 .UNSPECIFIED.,.F.,.F.,(4,4),(4.77362713684778,4.77483276840798),
 .UNSPECIFIED.);
#5870=B_SPLINE_CURVE_WITH_KNOTS('',3,(#24385,#24386,#24387,#24388,#24389,
#24390,#24391,#24392,#24393),.UNSPECIFIED.,.F.,.F.,(4,1,1,1,1,1,4),(4.69190485072485,
5.32399487973813,5.95608490875141,6.27212992325805,6.58817493776469,6.79887161410245,
6.9042290999944),.UNSPECIFIED.);
#5871=B_SPLINE_CURVE_WITH_KNOTS('',3,(#24394,#24395,#24396,#24397,#24398,
#24399,#24400,#24401,#24402,#24403),.UNSPECIFIED.,.F.,.F.,(4,1,1,1,1,1,
1,4),(6.90422178665282,7.00956829044021,7.22026496677796,7.43096164311572,
7.64165831945348,7.85235499579124,8.48444502480452,9.1165350538178),
 .UNSPECIFIED.);
#5872=B_SPLINE_CURVE_WITH_KNOTS('',3,(#24404,#24405,#24406,#24407),
 .UNSPECIFIED.,.F.,.F.,(4,4),(-9.03481070423354,-9.03360503529916),
 .UNSPECIFIED.);
#5873=B_SPLINE_CURVE_WITH_KNOTS('',3,(#24428,#24429,#24430,#24431,#24432,
#24433,#24434,#24435,#24436,#24437),.UNSPECIFIED.,.F.,.F.,(4,2,2,2,4),(-0.150488872007352,
-0.145598643293466,-0.0727993216467576,0.,0.00489022871386419),
 .UNSPECIFIED.);
#5874=B_SPLINE_CURVE_WITH_KNOTS('',3,(#24453,#24454,#24455,#24456,#24457,
#24458),.UNSPECIFIED.,.F.,.F.,(4,2,4),(1.30156425141723,1.60084152830946,
1.90011880520168),.UNSPECIFIED.);
#5875=B_SPLINE_CURVE_WITH_KNOTS('',3,(#24521,#24522,#24523,#24524,#24525,
#24526),.UNSPECIFIED.,.F.,.F.,(4,2,4),(0.,0.299277276892223,0.598554553784447),
 .UNSPECIFIED.);
#5876=B_SPLINE_CURVE_WITH_KNOTS('',3,(#24534,#24535,#24536,#24537,#24538,
#24539,#24540,#24541,#24542,#24543),.UNSPECIFIED.,.F.,.F.,(4,2,2,2,4),(-0.150488872007919,
-0.145598643294013,-0.0727993216470067,0.,0.00489022871390594),
 .UNSPECIFIED.);
#6709=VERTEX_POINT('',#22944);
#6710=VERTEX_POINT('',#22945);
#6711=VERTEX_POINT('',#22954);
#6712=VERTEX_POINT('',#22956);
#6713=VERTEX_POINT('',#22960);
#6714=VERTEX_POINT('',#22962);
#6715=VERTEX_POINT('',#22971);
#6716=VERTEX_POINT('',#22973);
#6717=VERTEX_POINT('',#22975);
#6718=VERTEX_POINT('',#22979);
#6719=VERTEX_POINT('',#22981);
#6720=VERTEX_POINT('',#22983);
#6721=VERTEX_POINT('',#22994);
#6722=VERTEX_POINT('',#23003);
#6723=VERTEX_POINT('',#23007);
#6724=VERTEX_POINT('',#23009);
#6725=VERTEX_POINT('',#23015);
#6726=VERTEX_POINT('',#23016);
#6727=VERTEX_POINT('',#23025);
#6728=VERTEX_POINT('',#23027);
#6729=VERTEX_POINT('',#23031);
#6730=VERTEX_POINT('',#23033);
#6731=VERTEX_POINT('',#23042);
#6732=VERTEX_POINT('',#23044);
#6733=VERTEX_POINT('',#23046);
#6734=VERTEX_POINT('',#23050);
#6735=VERTEX_POINT('',#23052);
#6736=VERTEX_POINT('',#23054);
#6737=VERTEX_POINT('',#23065);
#6738=VERTEX_POINT('',#23074);
#6739=VERTEX_POINT('',#23078);
#6740=VERTEX_POINT('',#23080);
#6741=VERTEX_POINT('',#23086);
#6742=VERTEX_POINT('',#23090);
#6743=VERTEX_POINT('',#23091);
#6744=VERTEX_POINT('',#23093);
#6745=VERTEX_POINT('',#23095);
#6746=VERTEX_POINT('',#23097);
#6747=VERTEX_POINT('',#23099);
#6748=VERTEX_POINT('',#23101);
#6749=VERTEX_POINT('',#23103);
#6750=VERTEX_POINT('',#23106);
#6751=VERTEX_POINT('',#23108);
#6752=VERTEX_POINT('',#23113);
#6753=VERTEX_POINT('',#23115);
#6754=VERTEX_POINT('',#23119);
#6755=VERTEX_POINT('',#23120);
#6756=VERTEX_POINT('',#23122);
#6757=VERTEX_POINT('',#23124);
#6758=VERTEX_POINT('',#23126);
#6759=VERTEX_POINT('',#23128);
#6760=VERTEX_POINT('',#23130);
#6761=VERTEX_POINT('',#23132);
#6762=VERTEX_POINT('',#23135);
#6763=VERTEX_POINT('',#23137);
#6764=VERTEX_POINT('',#23140);
#6765=VERTEX_POINT('',#23144);
#6766=VERTEX_POINT('',#23148);
#6767=VERTEX_POINT('',#23152);
#6768=VERTEX_POINT('',#23153);
#6769=VERTEX_POINT('',#23162);
#6770=VERTEX_POINT('',#23164);
#6771=VERTEX_POINT('',#23179);
#6772=VERTEX_POINT('',#23186);
#6773=VERTEX_POINT('',#23188);
#6774=VERTEX_POINT('',#23195);
#6775=VERTEX_POINT('',#23204);
#6776=VERTEX_POINT('',#23205);
#6777=VERTEX_POINT('',#23214);
#6778=VERTEX_POINT('',#23216);
#6779=VERTEX_POINT('',#23225);
#6780=VERTEX_POINT('',#23229);
#6781=VERTEX_POINT('',#23234);
#6782=VERTEX_POINT('',#23238);
#6783=VERTEX_POINT('',#23245);
#6784=VERTEX_POINT('',#23258);
#6785=VERTEX_POINT('',#23260);
#6786=VERTEX_POINT('',#23262);
#6787=VERTEX_POINT('',#23267);
#6788=VERTEX_POINT('',#23283);
#6789=VERTEX_POINT('',#23299);
#6790=VERTEX_POINT('',#23314);
#6791=VERTEX_POINT('',#23332);
#6792=VERTEX_POINT('',#23333);
#6793=VERTEX_POINT('',#23335);
#6794=VERTEX_POINT('',#23337);
#6795=VERTEX_POINT('',#23340);
#6796=VERTEX_POINT('',#23341);
#6797=VERTEX_POINT('',#23343);
#6798=VERTEX_POINT('',#23345);
#6799=VERTEX_POINT('',#23348);
#6800=VERTEX_POINT('',#23349);
#6801=VERTEX_POINT('',#23351);
#6802=VERTEX_POINT('',#23353);
#6803=VERTEX_POINT('',#23356);
#6804=VERTEX_POINT('',#23357);
#6805=VERTEX_POINT('',#23359);
#6806=VERTEX_POINT('',#23361);
#6807=VERTEX_POINT('',#23364);
#6808=VERTEX_POINT('',#23365);
#6809=VERTEX_POINT('',#23367);
#6810=VERTEX_POINT('',#23369);
#6811=VERTEX_POINT('',#23372);
#6812=VERTEX_POINT('',#23373);
#6813=VERTEX_POINT('',#23375);
#6814=VERTEX_POINT('',#23377);
#6815=VERTEX_POINT('',#23381);
#6816=VERTEX_POINT('',#23382);
#6817=VERTEX_POINT('',#23393);
#6818=VERTEX_POINT('',#23395);
#6819=VERTEX_POINT('',#23400);
#6820=VERTEX_POINT('',#23413);
#6821=VERTEX_POINT('',#23422);
#6822=VERTEX_POINT('',#23425);
#6823=VERTEX_POINT('',#23427);
#6824=VERTEX_POINT('',#23433);
#6825=VERTEX_POINT('',#23435);
#6826=VERTEX_POINT('',#23437);
#6827=VERTEX_POINT('',#23440);
#6828=VERTEX_POINT('',#23449);
#6829=VERTEX_POINT('',#23451);
#6830=VERTEX_POINT('',#23460);
#6831=VERTEX_POINT('',#23465);
#6832=VERTEX_POINT('',#23472);
#6833=VERTEX_POINT('',#23474);
#6834=VERTEX_POINT('',#23481);
#6835=VERTEX_POINT('',#23486);
#6836=VERTEX_POINT('',#23488);
#6837=VERTEX_POINT('',#23495);
#6838=VERTEX_POINT('',#23503);
#6839=VERTEX_POINT('',#23507);
#6840=VERTEX_POINT('',#23508);
#6841=VERTEX_POINT('',#23513);
#6842=VERTEX_POINT('',#23515);
#6843=VERTEX_POINT('',#23526);
#6844=VERTEX_POINT('',#23537);
#6845=VERTEX_POINT('',#23542);
#6846=VERTEX_POINT('',#23545);
#6847=VERTEX_POINT('',#23547);
#6848=VERTEX_POINT('',#23557);
#6849=VERTEX_POINT('',#23559);
#6850=VERTEX_POINT('',#23561);
#6851=VERTEX_POINT('',#23581);
#6852=VERTEX_POINT('',#23585);
#6853=VERTEX_POINT('',#23587);
#6854=VERTEX_POINT('',#23589);
#6855=VERTEX_POINT('',#23591);
#6856=VERTEX_POINT('',#23593);
#6857=VERTEX_POINT('',#23595);
#6858=VERTEX_POINT('',#23597);
#6859=VERTEX_POINT('',#23600);
#6860=VERTEX_POINT('',#23602);
#6861=VERTEX_POINT('',#23606);
#6862=VERTEX_POINT('',#23607);
#6863=VERTEX_POINT('',#23612);
#6864=VERTEX_POINT('',#23613);
#6865=VERTEX_POINT('',#23618);
#6866=VERTEX_POINT('',#23619);
#6867=VERTEX_POINT('',#23630);
#6868=VERTEX_POINT('',#23632);
#6869=VERTEX_POINT('',#23634);
#6870=VERTEX_POINT('',#23636);
#6871=VERTEX_POINT('',#23640);
#6872=VERTEX_POINT('',#23642);
#6873=VERTEX_POINT('',#23649);
#6874=VERTEX_POINT('',#23653);
#6875=VERTEX_POINT('',#23657);
#6876=VERTEX_POINT('',#23661);
#6877=VERTEX_POINT('',#23665);
#6878=VERTEX_POINT('',#23669);
#6879=VERTEX_POINT('',#23675);
#6880=VERTEX_POINT('',#23680);
#6881=VERTEX_POINT('',#23686);
#6882=VERTEX_POINT('',#23688);
#6883=VERTEX_POINT('',#23697);
#6884=VERTEX_POINT('',#23699);
#6885=VERTEX_POINT('',#23707);
#6886=VERTEX_POINT('',#23709);
#6887=VERTEX_POINT('',#23713);
#6888=VERTEX_POINT('',#23715);
#6889=VERTEX_POINT('',#23719);
#6890=VERTEX_POINT('',#23820);
#6891=VERTEX_POINT('',#23821);
#6892=VERTEX_POINT('',#23967);
#6893=VERTEX_POINT('',#23972);
#6894=VERTEX_POINT('',#23983);
#6895=VERTEX_POINT('',#23993);
#6896=VERTEX_POINT('',#24003);
#6897=VERTEX_POINT('',#24052);
#6898=VERTEX_POINT('',#24054);
#6899=VERTEX_POINT('',#24059);
#6900=VERTEX_POINT('',#24061);
#6901=VERTEX_POINT('',#24110);
#6902=VERTEX_POINT('',#24111);
#6903=VERTEX_POINT('',#24117);
#6904=VERTEX_POINT('',#24119);
#6905=VERTEX_POINT('',#24239);
#6906=VERTEX_POINT('',#24240);
#6907=VERTEX_POINT('',#24384);
#6908=VERTEX_POINT('',#24409);
#6909=VERTEX_POINT('',#24413);
#6910=VERTEX_POINT('',#24416);
#6911=VERTEX_POINT('',#24420);
#6912=VERTEX_POINT('',#24422);
#6913=VERTEX_POINT('',#24426);
#6914=VERTEX_POINT('',#24427);
#6915=VERTEX_POINT('',#24439);
#6916=VERTEX_POINT('',#24441);
#6917=VERTEX_POINT('',#24445);
#6918=VERTEX_POINT('',#24446);
#6919=VERTEX_POINT('',#24451);
#6920=VERTEX_POINT('',#24452);
#6921=VERTEX_POINT('',#24462);
#6922=VERTEX_POINT('',#24464);
#6923=VERTEX_POINT('',#24468);
#6924=VERTEX_POINT('',#24477);
#6925=VERTEX_POINT('',#24479);
#6926=VERTEX_POINT('',#24483);
#6927=VERTEX_POINT('',#24487);
#6928=VERTEX_POINT('',#24498);
#6929=VERTEX_POINT('',#24506);
#6930=VERTEX_POINT('',#24508);
#6931=VERTEX_POINT('',#24513);
#6932=VERTEX_POINT('',#24517);
#6933=VERTEX_POINT('',#24519);
#6934=VERTEX_POINT('',#24528);
#6935=VERTEX_POINT('',#24532);
#6936=VERTEX_POINT('',#24533);
#6937=VERTEX_POINT('',#24545);
#6938=VERTEX_POINT('',#24547);
#6939=VERTEX_POINT('',#24609);
#6940=VERTEX_POINT('',#24613);
#6941=VERTEX_POINT('',#24616);
#6942=VERTEX_POINT('',#24621);
#8289=EDGE_CURVE('',#6709,#6710,#5809,.F.);
#8290=EDGE_CURVE('',#6710,#6711,#3901,.T.);
#8291=EDGE_CURVE('',#6711,#6712,#3902,.F.);
#8292=EDGE_CURVE('',#6712,#6709,#3903,.T.);
#8293=EDGE_CURVE('',#6713,#6711,#3904,.T.);
#8294=EDGE_CURVE('',#6710,#6714,#5810,.T.);
#8295=EDGE_CURVE('',#6714,#6715,#3905,.T.);
#8296=EDGE_CURVE('',#6715,#6716,#3906,.T.);
#8297=EDGE_CURVE('',#6717,#6716,#1761,.T.);
#8298=EDGE_CURVE('',#6718,#6717,#3907,.T.);
#8299=EDGE_CURVE('',#6718,#6719,#3908,.T.);
#8300=EDGE_CURVE('',#6720,#6719,#5811,.F.);
#8301=EDGE_CURVE('',#6713,#6720,#3909,.T.);
#8302=EDGE_CURVE('',#6720,#6721,#5812,.F.);
#8303=EDGE_CURVE('',#6721,#6722,#3910,.T.);
#8304=EDGE_CURVE('',#6722,#6713,#3911,.F.);
#8305=EDGE_CURVE('',#6723,#6723,#662,.T.);
#8306=EDGE_CURVE('',#6723,#6724,#3912,.T.);
#8307=EDGE_CURVE('',#6709,#6724,#663,.T.);
#8308=EDGE_CURVE('',#6712,#6722,#664,.T.);
#8309=EDGE_CURVE('',#6724,#6721,#665,.T.);
#8310=EDGE_CURVE('',#6725,#6726,#5813,.F.);
#8311=EDGE_CURVE('',#6726,#6727,#3913,.T.);
#8312=EDGE_CURVE('',#6727,#6728,#3914,.F.);
#8313=EDGE_CURVE('',#6728,#6725,#3915,.T.);
#8314=EDGE_CURVE('',#6729,#6727,#3916,.T.);
#8315=EDGE_CURVE('',#6726,#6730,#5814,.T.);
#8316=EDGE_CURVE('',#6730,#6731,#3917,.T.);
#8317=EDGE_CURVE('',#6731,#6732,#3918,.T.);
#8318=EDGE_CURVE('',#6733,#6732,#1762,.T.);
#8319=EDGE_CURVE('',#6734,#6733,#3919,.T.);
#8320=EDGE_CURVE('',#6734,#6735,#3920,.T.);
#8321=EDGE_CURVE('',#6736,#6735,#5815,.F.);
#8322=EDGE_CURVE('',#6729,#6736,#3921,.T.);
#8323=EDGE_CURVE('',#6736,#6737,#5816,.F.);
#8324=EDGE_CURVE('',#6737,#6738,#3922,.T.);
#8325=EDGE_CURVE('',#6738,#6729,#3923,.F.);
#8326=EDGE_CURVE('',#6739,#6739,#666,.T.);
#8327=EDGE_CURVE('',#6739,#6740,#3924,.T.);
#8328=EDGE_CURVE('',#6725,#6740,#667,.T.);
#8329=EDGE_CURVE('',#6728,#6738,#668,.T.);
#8330=EDGE_CURVE('',#6740,#6737,#669,.T.);
#8331=EDGE_CURVE('',#6741,#6741,#670,.T.);
#8332=EDGE_CURVE('',#6741,#6723,#3925,.T.);
#8333=EDGE_CURVE('',#6742,#6743,#671,.T.);
#8334=EDGE_CURVE('',#6744,#6742,#3926,.T.);
#8335=EDGE_CURVE('',#6745,#6744,#672,.T.);
#8336=EDGE_CURVE('',#6746,#6745,#3927,.T.);
#8337=EDGE_CURVE('',#6747,#6746,#673,.T.);
#8338=EDGE_CURVE('',#6748,#6747,#3928,.T.);
#8339=EDGE_CURVE('',#6749,#6748,#674,.T.);
#8340=EDGE_CURVE('',#6743,#6749,#3929,.T.);
#8341=EDGE_CURVE('',#6750,#6750,#675,.T.);
#8342=EDGE_CURVE('',#6751,#6751,#676,.T.);
#8343=EDGE_CURVE('',#6750,#6739,#3930,.T.);
#8344=EDGE_CURVE('',#6752,#6752,#677,.T.);
#8345=EDGE_CURVE('',#6752,#6753,#3931,.T.);
#8346=EDGE_CURVE('',#6753,#6753,#678,.T.);
#8347=EDGE_CURVE('',#6754,#6755,#3932,.T.);
#8348=EDGE_CURVE('',#6756,#6754,#679,.T.);
#8349=EDGE_CURVE('',#6757,#6756,#3933,.T.);
#8350=EDGE_CURVE('',#6758,#6757,#680,.T.);
#8351=EDGE_CURVE('',#6759,#6758,#3934,.T.);
#8352=EDGE_CURVE('',#6760,#6759,#681,.T.);
#8353=EDGE_CURVE('',#6761,#6760,#3935,.T.);
#8354=EDGE_CURVE('',#6755,#6761,#682,.T.);
#8355=EDGE_CURVE('',#6762,#6762,#683,.T.);
#8356=EDGE_CURVE('',#6763,#6763,#684,.T.);
#8357=EDGE_CURVE('',#6753,#6764,#3936,.T.);
#8358=EDGE_CURVE('',#6764,#6764,#685,.T.);
#8359=EDGE_CURVE('',#6762,#6765,#3937,.T.);
#8360=EDGE_CURVE('',#6765,#6765,#686,.T.);
#8361=EDGE_CURVE('',#6765,#6766,#3938,.T.);
#8362=EDGE_CURVE('',#6766,#6766,#687,.T.);
#8363=EDGE_CURVE('',#6767,#6768,#5817,.F.);
#8364=EDGE_CURVE('',#6768,#6769,#688,.T.);
#8365=EDGE_CURVE('',#6769,#6770,#5818,.F.);
#8366=EDGE_CURVE('',#6770,#6767,#689,.T.);
#8367=EDGE_CURVE('',#6768,#6717,#5819,.T.);
#8368=EDGE_CURVE('',#6716,#6771,#5820,.T.);
#8369=EDGE_CURVE('',#6771,#6772,#690,.T.);
#8370=EDGE_CURVE('',#6772,#6773,#5821,.T.);
#8371=EDGE_CURVE('',#6773,#6774,#1763,.T.);
#8372=EDGE_CURVE('',#6774,#6769,#5822,.T.);
#8373=EDGE_CURVE('',#6775,#6776,#5823,.F.);
#8374=EDGE_CURVE('',#6776,#6777,#691,.T.);
#8375=EDGE_CURVE('',#6777,#6778,#5824,.F.);
#8376=EDGE_CURVE('',#6778,#6779,#692,.T.);
#8377=EDGE_CURVE('',#6779,#6775,#693,.T.);
#8378=EDGE_CURVE('',#6776,#6780,#5825,.T.);
#8379=EDGE_CURVE('',#6780,#6781,#1764,.T.);
#8380=EDGE_CURVE('',#6781,#6782,#5826,.T.);
#8381=EDGE_CURVE('',#6782,#6783,#694,.T.);
#8382=EDGE_CURVE('',#6783,#6733,#5827,.T.);
#8383=EDGE_CURVE('',#6732,#6777,#5828,.T.);
#8384=EDGE_CURVE('',#6784,#6784,#695,.T.);
#8385=EDGE_CURVE('',#6784,#6785,#696,.T.);
#8386=EDGE_CURVE('',#6785,#6786,#697,.T.);
#8387=EDGE_CURVE('',#6786,#6785,#698,.T.);
#8388=EDGE_CURVE('',#6786,#6779,#3939,.T.);
#8389=EDGE_CURVE('',#6778,#6787,#5829,.T.);
#8390=EDGE_CURVE('',#6787,#6788,#699,.T.);
#8391=EDGE_CURVE('',#6788,#6767,#5830,.T.);
#8392=EDGE_CURVE('',#6770,#6789,#5831,.T.);
#8393=EDGE_CURVE('',#6789,#6790,#700,.T.);
#8394=EDGE_CURVE('',#6790,#6775,#5832,.T.);
#8395=EDGE_CURVE('',#6791,#6792,#3940,.T.);
#8396=EDGE_CURVE('',#6792,#6793,#3941,.T.);
#8397=EDGE_CURVE('',#6793,#6794,#3942,.T.);
#8398=EDGE_CURVE('',#6794,#6791,#3943,.T.);
#8399=EDGE_CURVE('',#6795,#6796,#3944,.T.);
#8400=EDGE_CURVE('',#6796,#6797,#3945,.T.);
#8401=EDGE_CURVE('',#6797,#6798,#3946,.T.);
#8402=EDGE_CURVE('',#6798,#6795,#3947,.T.);
#8403=EDGE_CURVE('',#6799,#6800,#3948,.T.);
#8404=EDGE_CURVE('',#6800,#6801,#3949,.T.);
#8405=EDGE_CURVE('',#6801,#6802,#3950,.T.);
#8406=EDGE_CURVE('',#6802,#6799,#3951,.T.);
#8407=EDGE_CURVE('',#6803,#6804,#3952,.T.);
#8408=EDGE_CURVE('',#6804,#6805,#3953,.T.);
#8409=EDGE_CURVE('',#6805,#6806,#3954,.T.);
#8410=EDGE_CURVE('',#6806,#6803,#3955,.T.);
#8411=EDGE_CURVE('',#6807,#6808,#3956,.T.);
#8412=EDGE_CURVE('',#6808,#6809,#3957,.T.);
#8413=EDGE_CURVE('',#6809,#6810,#3958,.T.);
#8414=EDGE_CURVE('',#6810,#6807,#3959,.T.);
#8415=EDGE_CURVE('',#6811,#6812,#3960,.T.);
#8416=EDGE_CURVE('',#6812,#6813,#3961,.T.);
#8417=EDGE_CURVE('',#6813,#6814,#3962,.T.);
#8418=EDGE_CURVE('',#6814,#6811,#3963,.T.);
#8419=EDGE_CURVE('',#6815,#6816,#5833,.F.);
#8420=EDGE_CURVE('',#6817,#6816,#701,.T.);
#8421=EDGE_CURVE('',#6817,#6818,#5834,.F.);
#8422=EDGE_CURVE('',#6819,#6818,#5835,.T.);
#8423=EDGE_CURVE('',#6819,#6815,#702,.T.);
#8424=EDGE_CURVE('',#6820,#6819,#5836,.F.);
#8425=EDGE_CURVE('',#6820,#6821,#3964,.T.);
#8426=EDGE_CURVE('',#6821,#6783,#3965,.T.);
#8427=EDGE_CURVE('',#6782,#6822,#3966,.T.);
#8428=EDGE_CURVE('',#6822,#6823,#3967,.T.);
#8429=EDGE_CURVE('',#6815,#6823,#5837,.F.);
#8430=EDGE_CURVE('',#6824,#6824,#703,.T.);
#8431=EDGE_CURVE('',#6825,#6825,#704,.T.);
#8432=EDGE_CURVE('',#6826,#6826,#705,.T.);
#8433=EDGE_CURVE('',#6816,#6827,#5838,.F.);
#8434=EDGE_CURVE('',#6827,#6828,#706,.T.);
#8435=EDGE_CURVE('',#6828,#6829,#707,.T.);
#8436=EDGE_CURVE('',#6829,#6817,#5839,.F.);
#8437=EDGE_CURVE('',#6830,#6827,#5840,.F.);
#8438=EDGE_CURVE('',#6830,#6831,#5841,.T.);
#8439=EDGE_CURVE('',#6831,#6832,#708,.T.);
#8440=EDGE_CURVE('',#6832,#6833,#5842,.T.);
#8441=EDGE_CURVE('',#6833,#6834,#5843,.T.);
#8442=EDGE_CURVE('',#6835,#6834,#709,.T.);
#8443=EDGE_CURVE('',#6835,#6836,#5844,.T.);
#8444=EDGE_CURVE('',#6836,#6837,#710,.T.);
#8445=EDGE_CURVE('',#6837,#6829,#5845,.T.);
#8446=EDGE_CURVE('',#6828,#6838,#3968,.T.);
#8447=EDGE_CURVE('',#6838,#6838,#711,.T.);
#8448=EDGE_CURVE('',#6839,#6840,#5846,.T.);
#8449=EDGE_CURVE('',#6841,#6839,#712,.T.);
#8450=EDGE_CURVE('',#6842,#6841,#5847,.T.);
#8451=EDGE_CURVE('',#6842,#6843,#713,.T.);
#8452=EDGE_CURVE('',#6843,#6840,#5848,.F.);
#8453=EDGE_CURVE('',#6842,#6844,#5849,.T.);
#8454=EDGE_CURVE('',#6844,#6845,#3969,.T.);
#8455=EDGE_CURVE('',#6845,#6772,#3970,.T.);
#8456=EDGE_CURVE('',#6771,#6846,#3971,.T.);
#8457=EDGE_CURVE('',#6846,#6847,#3972,.T.);
#8458=EDGE_CURVE('',#6847,#6843,#5850,.T.);
#8459=EDGE_CURVE('',#6848,#6848,#714,.T.);
#8460=EDGE_CURVE('',#6849,#6849,#715,.T.);
#8461=EDGE_CURVE('',#6850,#6850,#716,.T.);
#8462=EDGE_CURVE('',#6834,#6841,#5851,.F.);
#8463=EDGE_CURVE('',#6839,#6835,#5852,.F.);
#8464=EDGE_CURVE('',#6838,#6851,#717,.T.);
#8465=EDGE_CURVE('',#6851,#6851,#718,.T.);
#8466=EDGE_CURVE('',#6852,#6852,#719,.T.);
#8467=EDGE_CURVE('',#6853,#6853,#720,.T.);
#8468=EDGE_CURVE('',#6854,#6854,#721,.T.);
#8469=EDGE_CURVE('',#6855,#6855,#722,.T.);
#8470=EDGE_CURVE('',#6856,#6856,#723,.T.);
#8471=EDGE_CURVE('',#6857,#6857,#724,.T.);
#8472=EDGE_CURVE('',#6858,#6858,#725,.T.);
#8473=EDGE_CURVE('',#6823,#6859,#726,.T.);
#8474=EDGE_CURVE('',#6859,#6860,#727,.T.);
#8475=EDGE_CURVE('',#6860,#6830,#728,.T.);
#8476=EDGE_CURVE('',#6861,#6862,#729,.T.);
#8477=EDGE_CURVE('',#6862,#6860,#3973,.T.);
#8478=EDGE_CURVE('',#6859,#6861,#3974,.T.);
#8479=EDGE_CURVE('',#6863,#6864,#730,.T.);
#8480=EDGE_CURVE('',#6864,#6862,#731,.T.);
#8481=EDGE_CURVE('',#6861,#6863,#732,.T.);
#8482=EDGE_CURVE('',#6865,#6866,#5853,.F.);
#8483=EDGE_CURVE('',#6866,#6864,#3975,.T.);
#8484=EDGE_CURVE('',#6863,#6865,#3976,.T.);
#8485=EDGE_CURVE('',#6790,#6866,#3977,.T.);
#8486=EDGE_CURVE('',#6789,#6867,#3978,.T.);
#8487=EDGE_CURVE('',#6868,#6867,#3979,.T.);
#8488=EDGE_CURVE('',#6868,#6869,#3980,.T.);
#8489=EDGE_CURVE('',#6870,#6869,#3981,.T.);
#8490=EDGE_CURVE('',#6864,#6870,#3982,.T.);
#8491=EDGE_CURVE('',#6871,#6822,#733,.T.);
#8492=EDGE_CURVE('',#6872,#6871,#3983,.T.);
#8493=EDGE_CURVE('',#6865,#6872,#734,.T.);
#8494=EDGE_CURVE('',#6755,#6870,#735,.T.);
#8495=EDGE_CURVE('',#6869,#6754,#736,.T.);
#8496=EDGE_CURVE('',#6873,#6756,#737,.T.);
#8497=EDGE_CURVE('',#6869,#6873,#738,.T.);
#8498=EDGE_CURVE('',#6874,#6757,#739,.T.);
#8499=EDGE_CURVE('',#6873,#6874,#3984,.T.);
#8500=EDGE_CURVE('',#6875,#6758,#740,.T.);
#8501=EDGE_CURVE('',#6874,#6875,#741,.T.);
#8502=EDGE_CURVE('',#6876,#6759,#742,.T.);
#8503=EDGE_CURVE('',#6875,#6876,#3985,.T.);
#8504=EDGE_CURVE('',#6877,#6760,#743,.T.);
#8505=EDGE_CURVE('',#6876,#6877,#744,.T.);
#8506=EDGE_CURVE('',#6878,#6761,#745,.T.);
#8507=EDGE_CURVE('',#6877,#6878,#3986,.T.);
#8508=EDGE_CURVE('',#6878,#6870,#746,.T.);
#8509=EDGE_CURVE('',#6879,#6874,#3987,.T.);
#8510=EDGE_CURVE('',#6833,#6879,#747,.T.);
#8511=EDGE_CURVE('',#6832,#6875,#3988,.T.);
#8512=EDGE_CURVE('',#6880,#6873,#3989,.T.);
#8513=EDGE_CURVE('',#6879,#6880,#3990,.T.);
#8514=EDGE_CURVE('',#6880,#6868,#748,.T.);
#8515=EDGE_CURVE('',#6881,#6868,#749,.T.);
#8516=EDGE_CURVE('',#6867,#6882,#5854,.F.);
#8517=EDGE_CURVE('',#6882,#6881,#3991,.T.);
#8518=EDGE_CURVE('',#6880,#6883,#750,.T.);
#8519=EDGE_CURVE('',#6883,#6884,#3992,.T.);
#8520=EDGE_CURVE('',#6884,#6879,#751,.T.);
#8521=EDGE_CURVE('',#6884,#6844,#752,.T.);
#8522=EDGE_CURVE('',#6881,#6883,#753,.T.);
#8523=EDGE_CURVE('',#6885,#6882,#754,.T.);
#8524=EDGE_CURVE('',#6886,#6885,#3993,.T.);
#8525=EDGE_CURVE('',#6845,#6886,#755,.T.);
#8526=EDGE_CURVE('',#6858,#6887,#756,.T.);
#8527=EDGE_CURVE('',#6887,#6888,#757,.T.);
#8528=EDGE_CURVE('',#6888,#6887,#758,.T.);
#8529=EDGE_CURVE('',#6888,#6889,#3994,.T.);
#8530=EDGE_CURVE('',#6889,#6889,#759,.T.);
#8531=EDGE_CURVE('',#6890,#6891,#5855,.T.);
#8532=EDGE_CURVE('',#6891,#6892,#5856,.T.);
#8533=EDGE_CURVE('',#6892,#6893,#5857,.T.);
#8534=EDGE_CURVE('',#6893,#6894,#5858,.T.);
#8535=EDGE_CURVE('',#6894,#6895,#5859,.T.);
#8536=EDGE_CURVE('',#6895,#6896,#5860,.T.);
#8537=EDGE_CURVE('',#6896,#6890,#5861,.T.);
#8538=EDGE_CURVE('',#6897,#6893,#3995,.T.);
#8539=EDGE_CURVE('',#6892,#6898,#5862,.T.);
#8540=EDGE_CURVE('',#6898,#6899,#3996,.T.);
#8541=EDGE_CURVE('',#6899,#6900,#5863,.T.);
#8542=EDGE_CURVE('',#6897,#6900,#5864,.T.);
#8543=EDGE_CURVE('',#6901,#6902,#3997,.T.);
#8544=EDGE_CURVE('',#6902,#6896,#5865,.T.);
#8545=EDGE_CURVE('',#6895,#6903,#3998,.T.);
#8546=EDGE_CURVE('',#6903,#6904,#5866,.T.);
#8547=EDGE_CURVE('',#6904,#6901,#5867,.T.);
#8548=EDGE_CURVE('',#6905,#6906,#5868,.T.);
#8549=EDGE_CURVE('',#6904,#6906,#5869,.T.);
#8550=EDGE_CURVE('',#6903,#6907,#5870,.T.);
#8551=EDGE_CURVE('',#6907,#6897,#5871,.T.);
#8552=EDGE_CURVE('',#6900,#6905,#5872,.T.);
#8553=EDGE_CURVE('',#6908,#6898,#760,.T.);
#8554=EDGE_CURVE('',#6899,#6908,#761,.T.);
#8555=EDGE_CURVE('',#6909,#6909,#762,.T.);
#8556=EDGE_CURVE('',#6909,#6894,#3999,.T.);
#8557=EDGE_CURVE('',#6907,#6910,#4000,.T.);
#8558=EDGE_CURVE('',#6910,#6910,#763,.T.);
#8559=EDGE_CURVE('',#6818,#6911,#764,.T.);
#8560=EDGE_CURVE('',#6911,#6912,#765,.T.);
#8561=EDGE_CURVE('',#6912,#6820,#766,.T.);
#8562=EDGE_CURVE('',#6913,#6914,#5873,.T.);
#8563=EDGE_CURVE('',#6914,#6912,#4001,.T.);
#8564=EDGE_CURVE('',#6911,#6915,#4002,.T.);
#8565=EDGE_CURVE('',#6915,#6916,#767,.T.);
#8566=EDGE_CURVE('',#6916,#6913,#4003,.T.);
#8567=EDGE_CURVE('',#6917,#6918,#768,.T.);
#8568=EDGE_CURVE('',#6918,#6916,#769,.T.);
#8569=EDGE_CURVE('',#6915,#6917,#770,.T.);
#8570=EDGE_CURVE('',#6919,#6920,#5874,.F.);
#8571=EDGE_CURVE('',#6920,#6918,#4004,.T.);
#8572=EDGE_CURVE('',#6917,#6919,#4005,.T.);
#8573=EDGE_CURVE('',#6921,#6911,#4006,.T.);
#8574=EDGE_CURVE('',#6922,#6921,#4007,.T.);
#8575=EDGE_CURVE('',#6922,#6915,#4008,.T.);
#8576=EDGE_CURVE('',#6923,#6837,#4009,.T.);
#8577=EDGE_CURVE('',#6921,#6923,#771,.T.);
#8578=EDGE_CURVE('',#6735,#6914,#772,.T.);
#8579=EDGE_CURVE('',#6821,#6734,#773,.T.);
#8580=EDGE_CURVE('',#6913,#6730,#774,.T.);
#8581=EDGE_CURVE('',#6924,#6742,#775,.T.);
#8582=EDGE_CURVE('',#6743,#6925,#776,.T.);
#8583=EDGE_CURVE('',#6925,#6924,#777,.T.);
#8584=EDGE_CURVE('',#6749,#6926,#778,.T.);
#8585=EDGE_CURVE('',#6926,#6925,#4010,.T.);
#8586=EDGE_CURVE('',#6748,#6927,#779,.T.);
#8587=EDGE_CURVE('',#6927,#6926,#780,.T.);
#8588=EDGE_CURVE('',#6747,#6923,#781,.T.);
#8589=EDGE_CURVE('',#6923,#6927,#4011,.T.);
#8590=EDGE_CURVE('',#6746,#6921,#782,.T.);
#8591=EDGE_CURVE('',#6745,#6922,#783,.T.);
#8592=EDGE_CURVE('',#6744,#6928,#784,.T.);
#8593=EDGE_CURVE('',#6928,#6922,#785,.T.);
#8594=EDGE_CURVE('',#6924,#6928,#4012,.T.);
#8595=EDGE_CURVE('',#6928,#6917,#4013,.T.);
#8596=EDGE_CURVE('',#6924,#6929,#4014,.T.);
#8597=EDGE_CURVE('',#6930,#6929,#4015,.T.);
#8598=EDGE_CURVE('',#6930,#6788,#4016,.T.);
#8599=EDGE_CURVE('',#6919,#6787,#4017,.T.);
#8600=EDGE_CURVE('',#6925,#6931,#4018,.T.);
#8601=EDGE_CURVE('',#6929,#6931,#786,.T.);
#8602=EDGE_CURVE('',#6929,#6932,#787,.T.);
#8603=EDGE_CURVE('',#6932,#6933,#4019,.T.);
#8604=EDGE_CURVE('',#6933,#6930,#5875,.F.);
#8605=EDGE_CURVE('',#6931,#6934,#788,.T.);
#8606=EDGE_CURVE('',#6934,#6932,#789,.T.);
#8607=EDGE_CURVE('',#6935,#6936,#5876,.T.);
#8608=EDGE_CURVE('',#6936,#6934,#4020,.T.);
#8609=EDGE_CURVE('',#6931,#6937,#4021,.T.);
#8610=EDGE_CURVE('',#6937,#6938,#790,.T.);
#8611=EDGE_CURVE('',#6938,#6935,#4022,.T.);
#8612=EDGE_CURVE('',#6847,#6938,#791,.T.);
#8613=EDGE_CURVE('',#6937,#6840,#792,.T.);
#8614=EDGE_CURVE('',#6715,#6846,#793,.T.);
#8615=EDGE_CURVE('',#6935,#6714,#794,.T.);
#8616=EDGE_CURVE('',#6719,#6936,#795,.T.);
#8617=EDGE_CURVE('',#6933,#6718,#796,.T.);
#8618=EDGE_CURVE('',#6791,#6794,#797,.T.);
#8619=EDGE_CURVE('',#6793,#6792,#798,.T.);
#8620=EDGE_CURVE('',#6795,#6798,#799,.T.);
#8621=EDGE_CURVE('',#6797,#6796,#800,.T.);
#8622=EDGE_CURVE('',#6799,#6802,#801,.T.);
#8623=EDGE_CURVE('',#6801,#6800,#802,.T.);
#8624=EDGE_CURVE('',#6803,#6806,#803,.T.);
#8625=EDGE_CURVE('',#6805,#6804,#804,.T.);
#8626=EDGE_CURVE('',#6807,#6810,#805,.T.);
#8627=EDGE_CURVE('',#6809,#6808,#806,.T.);
#8628=EDGE_CURVE('',#6811,#6814,#807,.T.);
#8629=EDGE_CURVE('',#6813,#6812,#808,.T.);
#8630=EDGE_CURVE('',#6731,#6920,#809,.T.);
#8631=EDGE_CURVE('',#6852,#6826,#4023,.T.);
#8632=EDGE_CURVE('',#6853,#6850,#4024,.T.);
#8633=EDGE_CURVE('',#6854,#6849,#4025,.T.);
#8634=EDGE_CURVE('',#6855,#6825,#4026,.T.);
#8635=EDGE_CURVE('',#6856,#6824,#4027,.T.);
#8636=EDGE_CURVE('',#6857,#6848,#4028,.T.);
#8637=EDGE_CURVE('',#6751,#6939,#4029,.T.);
#8638=EDGE_CURVE('',#6939,#6939,#810,.T.);
#8639=EDGE_CURVE('',#6940,#6940,#811,.T.);
#8640=EDGE_CURVE('',#6940,#6941,#4030,.T.);
#8641=EDGE_CURVE('',#6941,#6941,#812,.T.);
#8642=EDGE_CURVE('',#6942,#6942,#813,.T.);
#8643=EDGE_CURVE('',#6942,#6763,#4031,.T.);
#8644=EDGE_CURVE('',#6889,#6908,#4032,.T.);
#8645=EDGE_CURVE('',#6902,#6901,#814,.T.);
#8646=EDGE_CURVE('',#6862,#6878,#4033,.T.);
#8647=EDGE_CURVE('',#6860,#6877,#4034,.T.);
#8648=EDGE_CURVE('',#6831,#6876,#4035,.T.);
#8649=EDGE_CURVE('',#6927,#6836,#4036,.T.);
#8650=EDGE_CURVE('',#6926,#6937,#4037,.T.);
#8651=EDGE_CURVE('',#6781,#6871,#4038,.T.);
#8652=EDGE_CURVE('',#6780,#6872,#4039,.T.);
#8653=EDGE_CURVE('',#6773,#6886,#4040,.T.);
#8654=EDGE_CURVE('',#6774,#6885,#4041,.T.);
#10764=ORIENTED_EDGE('',*,*,#8289,.T.);
#10765=ORIENTED_EDGE('',*,*,#8290,.T.);
#10766=ORIENTED_EDGE('',*,*,#8291,.T.);
#10767=ORIENTED_EDGE('',*,*,#8292,.T.);
#10768=ORIENTED_EDGE('',*,*,#8293,.T.);
#10769=ORIENTED_EDGE('',*,*,#8290,.F.);
#10770=ORIENTED_EDGE('',*,*,#8294,.T.);
#10771=ORIENTED_EDGE('',*,*,#8295,.T.);
#10772=ORIENTED_EDGE('',*,*,#8296,.T.);
#10773=ORIENTED_EDGE('',*,*,#8297,.F.);
#10774=ORIENTED_EDGE('',*,*,#8298,.F.);
#10775=ORIENTED_EDGE('',*,*,#8299,.T.);
#10776=ORIENTED_EDGE('',*,*,#8300,.F.);
#10777=ORIENTED_EDGE('',*,*,#8301,.F.);
#10778=ORIENTED_EDGE('',*,*,#8302,.T.);
#10779=ORIENTED_EDGE('',*,*,#8303,.T.);
#10780=ORIENTED_EDGE('',*,*,#8304,.T.);
#10781=ORIENTED_EDGE('',*,*,#8301,.T.);
#10782=ORIENTED_EDGE('',*,*,#8305,.F.);
#10783=ORIENTED_EDGE('',*,*,#8306,.T.);
#10784=ORIENTED_EDGE('',*,*,#8307,.F.);
#10785=ORIENTED_EDGE('',*,*,#8292,.F.);
#10786=ORIENTED_EDGE('',*,*,#8308,.T.);
#10787=ORIENTED_EDGE('',*,*,#8303,.F.);
#10788=ORIENTED_EDGE('',*,*,#8309,.F.);
#10789=ORIENTED_EDGE('',*,*,#8306,.F.);
#10790=ORIENTED_EDGE('',*,*,#8310,.T.);
#10791=ORIENTED_EDGE('',*,*,#8311,.T.);
#10792=ORIENTED_EDGE('',*,*,#8312,.T.);
#10793=ORIENTED_EDGE('',*,*,#8313,.T.);
#10794=ORIENTED_EDGE('',*,*,#8314,.T.);
#10795=ORIENTED_EDGE('',*,*,#8311,.F.);
#10796=ORIENTED_EDGE('',*,*,#8315,.T.);
#10797=ORIENTED_EDGE('',*,*,#8316,.T.);
#10798=ORIENTED_EDGE('',*,*,#8317,.T.);
#10799=ORIENTED_EDGE('',*,*,#8318,.F.);
#10800=ORIENTED_EDGE('',*,*,#8319,.F.);
#10801=ORIENTED_EDGE('',*,*,#8320,.T.);
#10802=ORIENTED_EDGE('',*,*,#8321,.F.);
#10803=ORIENTED_EDGE('',*,*,#8322,.F.);
#10804=ORIENTED_EDGE('',*,*,#8323,.T.);
#10805=ORIENTED_EDGE('',*,*,#8324,.T.);
#10806=ORIENTED_EDGE('',*,*,#8325,.T.);
#10807=ORIENTED_EDGE('',*,*,#8322,.T.);
#10808=ORIENTED_EDGE('',*,*,#8326,.F.);
#10809=ORIENTED_EDGE('',*,*,#8327,.T.);
#10810=ORIENTED_EDGE('',*,*,#8328,.F.);
#10811=ORIENTED_EDGE('',*,*,#8313,.F.);
#10812=ORIENTED_EDGE('',*,*,#8329,.T.);
#10813=ORIENTED_EDGE('',*,*,#8324,.F.);
#10814=ORIENTED_EDGE('',*,*,#8330,.F.);
#10815=ORIENTED_EDGE('',*,*,#8327,.F.);
#10816=ORIENTED_EDGE('',*,*,#8331,.T.);
#10817=ORIENTED_EDGE('',*,*,#8332,.T.);
#10818=ORIENTED_EDGE('',*,*,#8305,.T.);
#10819=ORIENTED_EDGE('',*,*,#8332,.F.);
#10820=ORIENTED_EDGE('',*,*,#8333,.F.);
#10821=ORIENTED_EDGE('',*,*,#8334,.F.);
#10822=ORIENTED_EDGE('',*,*,#8335,.F.);
#10823=ORIENTED_EDGE('',*,*,#8336,.F.);
#10824=ORIENTED_EDGE('',*,*,#8337,.F.);
#10825=ORIENTED_EDGE('',*,*,#8338,.F.);
#10826=ORIENTED_EDGE('',*,*,#8339,.F.);
#10827=ORIENTED_EDGE('',*,*,#8340,.F.);
#10828=ORIENTED_EDGE('',*,*,#8341,.F.);
#10829=ORIENTED_EDGE('',*,*,#8342,.T.);
#10830=ORIENTED_EDGE('',*,*,#8331,.F.);
#10831=ORIENTED_EDGE('',*,*,#8341,.T.);
#10832=ORIENTED_EDGE('',*,*,#8343,.T.);
#10833=ORIENTED_EDGE('',*,*,#8326,.T.);
#10834=ORIENTED_EDGE('',*,*,#8343,.F.);
#10835=ORIENTED_EDGE('',*,*,#8344,.T.);
#10836=ORIENTED_EDGE('',*,*,#8345,.T.);
#10837=ORIENTED_EDGE('',*,*,#8346,.T.);
#10838=ORIENTED_EDGE('',*,*,#8345,.F.);
#10839=ORIENTED_EDGE('',*,*,#8347,.F.);
#10840=ORIENTED_EDGE('',*,*,#8348,.F.);
#10841=ORIENTED_EDGE('',*,*,#8349,.F.);
#10842=ORIENTED_EDGE('',*,*,#8350,.F.);
#10843=ORIENTED_EDGE('',*,*,#8351,.F.);
#10844=ORIENTED_EDGE('',*,*,#8352,.F.);
#10845=ORIENTED_EDGE('',*,*,#8353,.F.);
#10846=ORIENTED_EDGE('',*,*,#8354,.F.);
#10847=ORIENTED_EDGE('',*,*,#8355,.F.);
#10848=ORIENTED_EDGE('',*,*,#8356,.T.);
#10849=ORIENTED_EDGE('',*,*,#8344,.F.);
#10850=ORIENTED_EDGE('',*,*,#8346,.F.);
#10851=ORIENTED_EDGE('',*,*,#8357,.T.);
#10852=ORIENTED_EDGE('',*,*,#8358,.T.);
#10853=ORIENTED_EDGE('',*,*,#8357,.F.);
#10854=ORIENTED_EDGE('',*,*,#8355,.T.);
#10855=ORIENTED_EDGE('',*,*,#8359,.T.);
#10856=ORIENTED_EDGE('',*,*,#8360,.T.);
#10857=ORIENTED_EDGE('',*,*,#8359,.F.);
#10858=ORIENTED_EDGE('',*,*,#8360,.F.);
#10859=ORIENTED_EDGE('',*,*,#8361,.T.);
#10860=ORIENTED_EDGE('',*,*,#8362,.T.);
#10861=ORIENTED_EDGE('',*,*,#8361,.F.);
#10862=ORIENTED_EDGE('',*,*,#8363,.T.);
#10863=ORIENTED_EDGE('',*,*,#8364,.T.);
#10864=ORIENTED_EDGE('',*,*,#8365,.T.);
#10865=ORIENTED_EDGE('',*,*,#8366,.T.);
#10866=ORIENTED_EDGE('',*,*,#8364,.F.);
#10867=ORIENTED_EDGE('',*,*,#8367,.T.);
#10868=ORIENTED_EDGE('',*,*,#8297,.T.);
#10869=ORIENTED_EDGE('',*,*,#8368,.T.);
#10870=ORIENTED_EDGE('',*,*,#8369,.T.);
#10871=ORIENTED_EDGE('',*,*,#8370,.T.);
#10872=ORIENTED_EDGE('',*,*,#8371,.T.);
#10873=ORIENTED_EDGE('',*,*,#8372,.T.);
#10874=ORIENTED_EDGE('',*,*,#8373,.T.);
#10875=ORIENTED_EDGE('',*,*,#8374,.T.);
#10876=ORIENTED_EDGE('',*,*,#8375,.T.);
#10877=ORIENTED_EDGE('',*,*,#8376,.T.);
#10878=ORIENTED_EDGE('',*,*,#8377,.T.);
#10879=ORIENTED_EDGE('',*,*,#8374,.F.);
#10880=ORIENTED_EDGE('',*,*,#8378,.T.);
#10881=ORIENTED_EDGE('',*,*,#8379,.T.);
#10882=ORIENTED_EDGE('',*,*,#8380,.T.);
#10883=ORIENTED_EDGE('',*,*,#8381,.T.);
#10884=ORIENTED_EDGE('',*,*,#8382,.T.);
#10885=ORIENTED_EDGE('',*,*,#8318,.T.);
#10886=ORIENTED_EDGE('',*,*,#8383,.T.);
#10887=ORIENTED_EDGE('',*,*,#8384,.T.);
#10888=ORIENTED_EDGE('',*,*,#8385,.T.);
#10889=ORIENTED_EDGE('',*,*,#8386,.T.);
#10890=ORIENTED_EDGE('',*,*,#8387,.T.);
#10891=ORIENTED_EDGE('',*,*,#8385,.F.);
#10892=ORIENTED_EDGE('',*,*,#8387,.F.);
#10893=ORIENTED_EDGE('',*,*,#8388,.T.);
#10894=ORIENTED_EDGE('',*,*,#8376,.F.);
#10895=ORIENTED_EDGE('',*,*,#8389,.T.);
#10896=ORIENTED_EDGE('',*,*,#8390,.T.);
#10897=ORIENTED_EDGE('',*,*,#8391,.T.);
#10898=ORIENTED_EDGE('',*,*,#8366,.F.);
#10899=ORIENTED_EDGE('',*,*,#8392,.T.);
#10900=ORIENTED_EDGE('',*,*,#8393,.T.);
#10901=ORIENTED_EDGE('',*,*,#8394,.T.);
#10902=ORIENTED_EDGE('',*,*,#8377,.F.);
#10903=ORIENTED_EDGE('',*,*,#8388,.F.);
#10904=ORIENTED_EDGE('',*,*,#8386,.F.);
#10905=ORIENTED_EDGE('',*,*,#8384,.F.);
#10906=ORIENTED_EDGE('',*,*,#8395,.T.);
#10907=ORIENTED_EDGE('',*,*,#8396,.T.);
#10908=ORIENTED_EDGE('',*,*,#8397,.T.);
#10909=ORIENTED_EDGE('',*,*,#8398,.T.);
#10910=ORIENTED_EDGE('',*,*,#8399,.T.);
#10911=ORIENTED_EDGE('',*,*,#8400,.T.);
#10912=ORIENTED_EDGE('',*,*,#8401,.T.);
#10913=ORIENTED_EDGE('',*,*,#8402,.T.);
#10914=ORIENTED_EDGE('',*,*,#8403,.T.);
#10915=ORIENTED_EDGE('',*,*,#8404,.T.);
#10916=ORIENTED_EDGE('',*,*,#8405,.T.);
#10917=ORIENTED_EDGE('',*,*,#8406,.T.);
#10918=ORIENTED_EDGE('',*,*,#8407,.T.);
#10919=ORIENTED_EDGE('',*,*,#8408,.T.);
#10920=ORIENTED_EDGE('',*,*,#8409,.T.);
#10921=ORIENTED_EDGE('',*,*,#8410,.T.);
#10922=ORIENTED_EDGE('',*,*,#8411,.T.);
#10923=ORIENTED_EDGE('',*,*,#8412,.T.);
#10924=ORIENTED_EDGE('',*,*,#8413,.T.);
#10925=ORIENTED_EDGE('',*,*,#8414,.T.);
#10926=ORIENTED_EDGE('',*,*,#8415,.T.);
#10927=ORIENTED_EDGE('',*,*,#8416,.T.);
#10928=ORIENTED_EDGE('',*,*,#8417,.T.);
#10929=ORIENTED_EDGE('',*,*,#8418,.T.);
#10930=ORIENTED_EDGE('',*,*,#8419,.T.);
#10931=ORIENTED_EDGE('',*,*,#8420,.F.);
#10932=ORIENTED_EDGE('',*,*,#8421,.T.);
#10933=ORIENTED_EDGE('',*,*,#8422,.F.);
#10934=ORIENTED_EDGE('',*,*,#8423,.T.);
#10935=ORIENTED_EDGE('',*,*,#8423,.F.);
#10936=ORIENTED_EDGE('',*,*,#8424,.F.);
#10937=ORIENTED_EDGE('',*,*,#8425,.T.);
#10938=ORIENTED_EDGE('',*,*,#8426,.T.);
#10939=ORIENTED_EDGE('',*,*,#8381,.F.);
#10940=ORIENTED_EDGE('',*,*,#8427,.T.);
#10941=ORIENTED_EDGE('',*,*,#8428,.T.);
#10942=ORIENTED_EDGE('',*,*,#8429,.F.);
#10943=ORIENTED_EDGE('',*,*,#8430,.T.);
#10944=ORIENTED_EDGE('',*,*,#8431,.T.);
#10945=ORIENTED_EDGE('',*,*,#8432,.T.);
#10946=ORIENTED_EDGE('',*,*,#8433,.T.);
#10947=ORIENTED_EDGE('',*,*,#8434,.T.);
#10948=ORIENTED_EDGE('',*,*,#8435,.T.);
#10949=ORIENTED_EDGE('',*,*,#8436,.T.);
#10950=ORIENTED_EDGE('',*,*,#8420,.T.);
#10951=ORIENTED_EDGE('',*,*,#8434,.F.);
#10952=ORIENTED_EDGE('',*,*,#8437,.F.);
#10953=ORIENTED_EDGE('',*,*,#8438,.T.);
#10954=ORIENTED_EDGE('',*,*,#8439,.T.);
#10955=ORIENTED_EDGE('',*,*,#8440,.T.);
#10956=ORIENTED_EDGE('',*,*,#8441,.T.);
#10957=ORIENTED_EDGE('',*,*,#8442,.F.);
#10958=ORIENTED_EDGE('',*,*,#8443,.T.);
#10959=ORIENTED_EDGE('',*,*,#8444,.T.);
#10960=ORIENTED_EDGE('',*,*,#8445,.T.);
#10961=ORIENTED_EDGE('',*,*,#8435,.F.);
#10962=ORIENTED_EDGE('',*,*,#8446,.T.);
#10963=ORIENTED_EDGE('',*,*,#8447,.F.);
#10964=ORIENTED_EDGE('',*,*,#8446,.F.);
#10965=ORIENTED_EDGE('',*,*,#8448,.F.);
#10966=ORIENTED_EDGE('',*,*,#8449,.F.);
#10967=ORIENTED_EDGE('',*,*,#8450,.F.);
#10968=ORIENTED_EDGE('',*,*,#8451,.T.);
#10969=ORIENTED_EDGE('',*,*,#8452,.T.);
#10970=ORIENTED_EDGE('',*,*,#8451,.F.);
#10971=ORIENTED_EDGE('',*,*,#8453,.T.);
#10972=ORIENTED_EDGE('',*,*,#8454,.T.);
#10973=ORIENTED_EDGE('',*,*,#8455,.T.);
#10974=ORIENTED_EDGE('',*,*,#8369,.F.);
#10975=ORIENTED_EDGE('',*,*,#8456,.T.);
#10976=ORIENTED_EDGE('',*,*,#8457,.T.);
#10977=ORIENTED_EDGE('',*,*,#8458,.T.);
#10978=ORIENTED_EDGE('',*,*,#8459,.T.);
#10979=ORIENTED_EDGE('',*,*,#8460,.T.);
#10980=ORIENTED_EDGE('',*,*,#8461,.T.);
#10981=ORIENTED_EDGE('',*,*,#8462,.T.);
#10982=ORIENTED_EDGE('',*,*,#8449,.T.);
#10983=ORIENTED_EDGE('',*,*,#8463,.T.);
#10984=ORIENTED_EDGE('',*,*,#8442,.T.);
#10985=ORIENTED_EDGE('',*,*,#8447,.T.);
#10986=ORIENTED_EDGE('',*,*,#8464,.T.);
#10987=ORIENTED_EDGE('',*,*,#8465,.T.);
#10988=ORIENTED_EDGE('',*,*,#8464,.F.);
#10989=ORIENTED_EDGE('',*,*,#8465,.F.);
#10990=ORIENTED_EDGE('',*,*,#8466,.T.);
#10991=ORIENTED_EDGE('',*,*,#8467,.T.);
#10992=ORIENTED_EDGE('',*,*,#8468,.T.);
#10993=ORIENTED_EDGE('',*,*,#8469,.T.);
#10994=ORIENTED_EDGE('',*,*,#8470,.T.);
#10995=ORIENTED_EDGE('',*,*,#8471,.T.);
#10996=ORIENTED_EDGE('',*,*,#8472,.F.);
#10997=ORIENTED_EDGE('',*,*,#8429,.T.);
#10998=ORIENTED_EDGE('',*,*,#8473,.T.);
#10999=ORIENTED_EDGE('',*,*,#8474,.T.);
#11000=ORIENTED_EDGE('',*,*,#8475,.T.);
#11001=ORIENTED_EDGE('',*,*,#8437,.T.);
#11002=ORIENTED_EDGE('',*,*,#8433,.F.);
#11003=ORIENTED_EDGE('',*,*,#8419,.F.);
#11004=ORIENTED_EDGE('',*,*,#8476,.T.);
#11005=ORIENTED_EDGE('',*,*,#8477,.T.);
#11006=ORIENTED_EDGE('',*,*,#8474,.F.);
#11007=ORIENTED_EDGE('',*,*,#8478,.T.);
#11008=ORIENTED_EDGE('',*,*,#8479,.T.);
#11009=ORIENTED_EDGE('',*,*,#8480,.T.);
#11010=ORIENTED_EDGE('',*,*,#8476,.F.);
#11011=ORIENTED_EDGE('',*,*,#8481,.T.);
#11012=ORIENTED_EDGE('',*,*,#8482,.T.);
#11013=ORIENTED_EDGE('',*,*,#8483,.T.);
#11014=ORIENTED_EDGE('',*,*,#8479,.F.);
#11015=ORIENTED_EDGE('',*,*,#8484,.T.);
#11016=ORIENTED_EDGE('',*,*,#8483,.F.);
#11017=ORIENTED_EDGE('',*,*,#8485,.F.);
#11018=ORIENTED_EDGE('',*,*,#8393,.F.);
#11019=ORIENTED_EDGE('',*,*,#8486,.T.);
#11020=ORIENTED_EDGE('',*,*,#8487,.F.);
#11021=ORIENTED_EDGE('',*,*,#8488,.T.);
#11022=ORIENTED_EDGE('',*,*,#8489,.F.);
#11023=ORIENTED_EDGE('',*,*,#8490,.F.);
#11024=ORIENTED_EDGE('',*,*,#8484,.F.);
#11025=ORIENTED_EDGE('',*,*,#8481,.F.);
#11026=ORIENTED_EDGE('',*,*,#8478,.F.);
#11027=ORIENTED_EDGE('',*,*,#8473,.F.);
#11028=ORIENTED_EDGE('',*,*,#8428,.F.);
#11029=ORIENTED_EDGE('',*,*,#8491,.F.);
#11030=ORIENTED_EDGE('',*,*,#8492,.F.);
#11031=ORIENTED_EDGE('',*,*,#8493,.F.);
#11032=ORIENTED_EDGE('',*,*,#8494,.T.);
#11033=ORIENTED_EDGE('',*,*,#8489,.T.);
#11034=ORIENTED_EDGE('',*,*,#8495,.T.);
#11035=ORIENTED_EDGE('',*,*,#8347,.T.);
#11036=ORIENTED_EDGE('',*,*,#8496,.T.);
#11037=ORIENTED_EDGE('',*,*,#8348,.T.);
#11038=ORIENTED_EDGE('',*,*,#8495,.F.);
#11039=ORIENTED_EDGE('',*,*,#8497,.T.);
#11040=ORIENTED_EDGE('',*,*,#8498,.T.);
#11041=ORIENTED_EDGE('',*,*,#8349,.T.);
#11042=ORIENTED_EDGE('',*,*,#8496,.F.);
#11043=ORIENTED_EDGE('',*,*,#8499,.T.);
#11044=ORIENTED_EDGE('',*,*,#8500,.T.);
#11045=ORIENTED_EDGE('',*,*,#8350,.T.);
#11046=ORIENTED_EDGE('',*,*,#8498,.F.);
#11047=ORIENTED_EDGE('',*,*,#8501,.T.);
#11048=ORIENTED_EDGE('',*,*,#8502,.T.);
#11049=ORIENTED_EDGE('',*,*,#8351,.T.);
#11050=ORIENTED_EDGE('',*,*,#8500,.F.);
#11051=ORIENTED_EDGE('',*,*,#8503,.T.);
#11052=ORIENTED_EDGE('',*,*,#8504,.T.);
#11053=ORIENTED_EDGE('',*,*,#8352,.T.);
#11054=ORIENTED_EDGE('',*,*,#8502,.F.);
#11055=ORIENTED_EDGE('',*,*,#8505,.T.);
#11056=ORIENTED_EDGE('',*,*,#8506,.T.);
#11057=ORIENTED_EDGE('',*,*,#8353,.T.);
#11058=ORIENTED_EDGE('',*,*,#8504,.F.);
#11059=ORIENTED_EDGE('',*,*,#8507,.T.);
#11060=ORIENTED_EDGE('',*,*,#8494,.F.);
#11061=ORIENTED_EDGE('',*,*,#8354,.T.);
#11062=ORIENTED_EDGE('',*,*,#8506,.F.);
#11063=ORIENTED_EDGE('',*,*,#8508,.T.);
#11064=ORIENTED_EDGE('',*,*,#8501,.F.);
#11065=ORIENTED_EDGE('',*,*,#8509,.F.);
#11066=ORIENTED_EDGE('',*,*,#8510,.F.);
#11067=ORIENTED_EDGE('',*,*,#8440,.F.);
#11068=ORIENTED_EDGE('',*,*,#8511,.T.);
#11069=ORIENTED_EDGE('',*,*,#8499,.F.);
#11070=ORIENTED_EDGE('',*,*,#8512,.F.);
#11071=ORIENTED_EDGE('',*,*,#8513,.F.);
#11072=ORIENTED_EDGE('',*,*,#8509,.T.);
#11073=ORIENTED_EDGE('',*,*,#8497,.F.);
#11074=ORIENTED_EDGE('',*,*,#8488,.F.);
#11075=ORIENTED_EDGE('',*,*,#8514,.F.);
#11076=ORIENTED_EDGE('',*,*,#8512,.T.);
#11077=ORIENTED_EDGE('',*,*,#8515,.T.);
#11078=ORIENTED_EDGE('',*,*,#8487,.T.);
#11079=ORIENTED_EDGE('',*,*,#8516,.T.);
#11080=ORIENTED_EDGE('',*,*,#8517,.T.);
#11081=ORIENTED_EDGE('',*,*,#8518,.T.);
#11082=ORIENTED_EDGE('',*,*,#8519,.T.);
#11083=ORIENTED_EDGE('',*,*,#8520,.T.);
#11084=ORIENTED_EDGE('',*,*,#8513,.T.);
#11085=ORIENTED_EDGE('',*,*,#8450,.T.);
#11086=ORIENTED_EDGE('',*,*,#8462,.F.);
#11087=ORIENTED_EDGE('',*,*,#8441,.F.);
#11088=ORIENTED_EDGE('',*,*,#8510,.T.);
#11089=ORIENTED_EDGE('',*,*,#8520,.F.);
#11090=ORIENTED_EDGE('',*,*,#8521,.T.);
#11091=ORIENTED_EDGE('',*,*,#8453,.F.);
#11092=ORIENTED_EDGE('',*,*,#8518,.F.);
#11093=ORIENTED_EDGE('',*,*,#8514,.T.);
#11094=ORIENTED_EDGE('',*,*,#8515,.F.);
#11095=ORIENTED_EDGE('',*,*,#8522,.T.);
#11096=ORIENTED_EDGE('',*,*,#8521,.F.);
#11097=ORIENTED_EDGE('',*,*,#8519,.F.);
#11098=ORIENTED_EDGE('',*,*,#8522,.F.);
#11099=ORIENTED_EDGE('',*,*,#8517,.F.);
#11100=ORIENTED_EDGE('',*,*,#8523,.F.);
#11101=ORIENTED_EDGE('',*,*,#8524,.F.);
#11102=ORIENTED_EDGE('',*,*,#8525,.F.);
#11103=ORIENTED_EDGE('',*,*,#8454,.F.);
#11104=ORIENTED_EDGE('',*,*,#8472,.T.);
#11105=ORIENTED_EDGE('',*,*,#8526,.T.);
#11106=ORIENTED_EDGE('',*,*,#8527,.T.);
#11107=ORIENTED_EDGE('',*,*,#8528,.T.);
#11108=ORIENTED_EDGE('',*,*,#8526,.F.);
#11109=ORIENTED_EDGE('',*,*,#8528,.F.);
#11110=ORIENTED_EDGE('',*,*,#8529,.T.);
#11111=ORIENTED_EDGE('',*,*,#8530,.T.);
#11112=ORIENTED_EDGE('',*,*,#8529,.F.);
#11113=ORIENTED_EDGE('',*,*,#8527,.F.);
#11114=ORIENTED_EDGE('',*,*,#8531,.T.);
#11115=ORIENTED_EDGE('',*,*,#8532,.T.);
#11116=ORIENTED_EDGE('',*,*,#8533,.T.);
#11117=ORIENTED_EDGE('',*,*,#8534,.T.);
#11118=ORIENTED_EDGE('',*,*,#8535,.T.);
#11119=ORIENTED_EDGE('',*,*,#8536,.T.);
#11120=ORIENTED_EDGE('',*,*,#8537,.T.);
#11121=ORIENTED_EDGE('',*,*,#8538,.T.);
#11122=ORIENTED_EDGE('',*,*,#8533,.F.);
#11123=ORIENTED_EDGE('',*,*,#8539,.T.);
#11124=ORIENTED_EDGE('',*,*,#8540,.T.);
#11125=ORIENTED_EDGE('',*,*,#8541,.T.);
#11126=ORIENTED_EDGE('',*,*,#8542,.F.);
#11127=ORIENTED_EDGE('',*,*,#8543,.T.);
#11128=ORIENTED_EDGE('',*,*,#8544,.T.);
#11129=ORIENTED_EDGE('',*,*,#8536,.F.);
#11130=ORIENTED_EDGE('',*,*,#8545,.T.);
#11131=ORIENTED_EDGE('',*,*,#8546,.T.);
#11132=ORIENTED_EDGE('',*,*,#8547,.T.);
#11133=ORIENTED_EDGE('',*,*,#8548,.T.);
#11134=ORIENTED_EDGE('',*,*,#8549,.F.);
#11135=ORIENTED_EDGE('',*,*,#8546,.F.);
#11136=ORIENTED_EDGE('',*,*,#8550,.T.);
#11137=ORIENTED_EDGE('',*,*,#8551,.T.);
#11138=ORIENTED_EDGE('',*,*,#8542,.T.);
#11139=ORIENTED_EDGE('',*,*,#8552,.T.);
#11140=ORIENTED_EDGE('',*,*,#8540,.F.);
#11141=ORIENTED_EDGE('',*,*,#8553,.F.);
#11142=ORIENTED_EDGE('',*,*,#8554,.F.);
#11143=ORIENTED_EDGE('',*,*,#8555,.F.);
#11144=ORIENTED_EDGE('',*,*,#8556,.T.);
#11145=ORIENTED_EDGE('',*,*,#8534,.F.);
#11146=ORIENTED_EDGE('',*,*,#8538,.F.);
#11147=ORIENTED_EDGE('',*,*,#8551,.F.);
#11148=ORIENTED_EDGE('',*,*,#8557,.T.);
#11149=ORIENTED_EDGE('',*,*,#8558,.T.);
#11150=ORIENTED_EDGE('',*,*,#8557,.F.);
#11151=ORIENTED_EDGE('',*,*,#8550,.F.);
#11152=ORIENTED_EDGE('',*,*,#8545,.F.);
#11153=ORIENTED_EDGE('',*,*,#8535,.F.);
#11154=ORIENTED_EDGE('',*,*,#8556,.F.);
#11155=ORIENTED_EDGE('',*,*,#8559,.T.);
#11156=ORIENTED_EDGE('',*,*,#8560,.T.);
#11157=ORIENTED_EDGE('',*,*,#8561,.T.);
#11158=ORIENTED_EDGE('',*,*,#8424,.T.);
#11159=ORIENTED_EDGE('',*,*,#8422,.T.);
#11160=ORIENTED_EDGE('',*,*,#8562,.T.);
#11161=ORIENTED_EDGE('',*,*,#8563,.T.);
#11162=ORIENTED_EDGE('',*,*,#8560,.F.);
#11163=ORIENTED_EDGE('',*,*,#8564,.T.);
#11164=ORIENTED_EDGE('',*,*,#8565,.T.);
#11165=ORIENTED_EDGE('',*,*,#8566,.T.);
#11166=ORIENTED_EDGE('',*,*,#8567,.T.);
#11167=ORIENTED_EDGE('',*,*,#8568,.T.);
#11168=ORIENTED_EDGE('',*,*,#8565,.F.);
#11169=ORIENTED_EDGE('',*,*,#8569,.T.);
#11170=ORIENTED_EDGE('',*,*,#8570,.T.);
#11171=ORIENTED_EDGE('',*,*,#8571,.T.);
#11172=ORIENTED_EDGE('',*,*,#8567,.F.);
#11173=ORIENTED_EDGE('',*,*,#8572,.T.);
#11174=ORIENTED_EDGE('',*,*,#8564,.F.);
#11175=ORIENTED_EDGE('',*,*,#8573,.F.);
#11176=ORIENTED_EDGE('',*,*,#8574,.F.);
#11177=ORIENTED_EDGE('',*,*,#8575,.T.);
#11178=ORIENTED_EDGE('',*,*,#8559,.F.);
#11179=ORIENTED_EDGE('',*,*,#8421,.F.);
#11180=ORIENTED_EDGE('',*,*,#8436,.F.);
#11181=ORIENTED_EDGE('',*,*,#8445,.F.);
#11182=ORIENTED_EDGE('',*,*,#8576,.F.);
#11183=ORIENTED_EDGE('',*,*,#8577,.F.);
#11184=ORIENTED_EDGE('',*,*,#8573,.T.);
#11185=ORIENTED_EDGE('',*,*,#8561,.F.);
#11186=ORIENTED_EDGE('',*,*,#8563,.F.);
#11187=ORIENTED_EDGE('',*,*,#8578,.F.);
#11188=ORIENTED_EDGE('',*,*,#8320,.F.);
#11189=ORIENTED_EDGE('',*,*,#8579,.F.);
#11190=ORIENTED_EDGE('',*,*,#8425,.F.);
#11191=ORIENTED_EDGE('',*,*,#8562,.F.);
#11192=ORIENTED_EDGE('',*,*,#8580,.T.);
#11193=ORIENTED_EDGE('',*,*,#8315,.F.);
#11194=ORIENTED_EDGE('',*,*,#8310,.F.);
#11195=ORIENTED_EDGE('',*,*,#8328,.T.);
#11196=ORIENTED_EDGE('',*,*,#8330,.T.);
#11197=ORIENTED_EDGE('',*,*,#8323,.F.);
#11198=ORIENTED_EDGE('',*,*,#8321,.T.);
#11199=ORIENTED_EDGE('',*,*,#8578,.T.);
#11200=ORIENTED_EDGE('',*,*,#8581,.T.);
#11201=ORIENTED_EDGE('',*,*,#8333,.T.);
#11202=ORIENTED_EDGE('',*,*,#8582,.T.);
#11203=ORIENTED_EDGE('',*,*,#8583,.T.);
#11204=ORIENTED_EDGE('',*,*,#8584,.T.);
#11205=ORIENTED_EDGE('',*,*,#8585,.T.);
#11206=ORIENTED_EDGE('',*,*,#8582,.F.);
#11207=ORIENTED_EDGE('',*,*,#8340,.T.);
#11208=ORIENTED_EDGE('',*,*,#8586,.T.);
#11209=ORIENTED_EDGE('',*,*,#8587,.T.);
#11210=ORIENTED_EDGE('',*,*,#8584,.F.);
#11211=ORIENTED_EDGE('',*,*,#8339,.T.);
#11212=ORIENTED_EDGE('',*,*,#8588,.T.);
#11213=ORIENTED_EDGE('',*,*,#8589,.T.);
#11214=ORIENTED_EDGE('',*,*,#8586,.F.);
#11215=ORIENTED_EDGE('',*,*,#8338,.T.);
#11216=ORIENTED_EDGE('',*,*,#8590,.T.);
#11217=ORIENTED_EDGE('',*,*,#8577,.T.);
#11218=ORIENTED_EDGE('',*,*,#8588,.F.);
#11219=ORIENTED_EDGE('',*,*,#8337,.T.);
#11220=ORIENTED_EDGE('',*,*,#8591,.T.);
#11221=ORIENTED_EDGE('',*,*,#8574,.T.);
#11222=ORIENTED_EDGE('',*,*,#8590,.F.);
#11223=ORIENTED_EDGE('',*,*,#8336,.T.);
#11224=ORIENTED_EDGE('',*,*,#8592,.T.);
#11225=ORIENTED_EDGE('',*,*,#8593,.T.);
#11226=ORIENTED_EDGE('',*,*,#8591,.F.);
#11227=ORIENTED_EDGE('',*,*,#8335,.T.);
#11228=ORIENTED_EDGE('',*,*,#8581,.F.);
#11229=ORIENTED_EDGE('',*,*,#8594,.T.);
#11230=ORIENTED_EDGE('',*,*,#8592,.F.);
#11231=ORIENTED_EDGE('',*,*,#8334,.T.);
#11232=ORIENTED_EDGE('',*,*,#8569,.F.);
#11233=ORIENTED_EDGE('',*,*,#8575,.F.);
#11234=ORIENTED_EDGE('',*,*,#8593,.F.);
#11235=ORIENTED_EDGE('',*,*,#8595,.T.);
#11236=ORIENTED_EDGE('',*,*,#8572,.F.);
#11237=ORIENTED_EDGE('',*,*,#8595,.F.);
#11238=ORIENTED_EDGE('',*,*,#8594,.F.);
#11239=ORIENTED_EDGE('',*,*,#8596,.T.);
#11240=ORIENTED_EDGE('',*,*,#8597,.F.);
#11241=ORIENTED_EDGE('',*,*,#8598,.T.);
#11242=ORIENTED_EDGE('',*,*,#8390,.F.);
#11243=ORIENTED_EDGE('',*,*,#8599,.F.);
#11244=ORIENTED_EDGE('',*,*,#8583,.F.);
#11245=ORIENTED_EDGE('',*,*,#8600,.T.);
#11246=ORIENTED_EDGE('',*,*,#8601,.F.);
#11247=ORIENTED_EDGE('',*,*,#8596,.F.);
#11248=ORIENTED_EDGE('',*,*,#8602,.T.);
#11249=ORIENTED_EDGE('',*,*,#8603,.T.);
#11250=ORIENTED_EDGE('',*,*,#8604,.T.);
#11251=ORIENTED_EDGE('',*,*,#8597,.T.);
#11252=ORIENTED_EDGE('',*,*,#8605,.T.);
#11253=ORIENTED_EDGE('',*,*,#8606,.T.);
#11254=ORIENTED_EDGE('',*,*,#8602,.F.);
#11255=ORIENTED_EDGE('',*,*,#8601,.T.);
#11256=ORIENTED_EDGE('',*,*,#8607,.T.);
#11257=ORIENTED_EDGE('',*,*,#8608,.T.);
#11258=ORIENTED_EDGE('',*,*,#8605,.F.);
#11259=ORIENTED_EDGE('',*,*,#8609,.T.);
#11260=ORIENTED_EDGE('',*,*,#8610,.T.);
#11261=ORIENTED_EDGE('',*,*,#8611,.T.);
#11262=ORIENTED_EDGE('',*,*,#8458,.F.);
#11263=ORIENTED_EDGE('',*,*,#8612,.T.);
#11264=ORIENTED_EDGE('',*,*,#8610,.F.);
#11265=ORIENTED_EDGE('',*,*,#8613,.T.);
#11266=ORIENTED_EDGE('',*,*,#8452,.F.);
#11267=ORIENTED_EDGE('',*,*,#8612,.F.);
#11268=ORIENTED_EDGE('',*,*,#8457,.F.);
#11269=ORIENTED_EDGE('',*,*,#8614,.F.);
#11270=ORIENTED_EDGE('',*,*,#8295,.F.);
#11271=ORIENTED_EDGE('',*,*,#8615,.F.);
#11272=ORIENTED_EDGE('',*,*,#8611,.F.);
#11273=ORIENTED_EDGE('',*,*,#8603,.F.);
#11274=ORIENTED_EDGE('',*,*,#8606,.F.);
#11275=ORIENTED_EDGE('',*,*,#8608,.F.);
#11276=ORIENTED_EDGE('',*,*,#8616,.F.);
#11277=ORIENTED_EDGE('',*,*,#8299,.F.);
#11278=ORIENTED_EDGE('',*,*,#8617,.F.);
#11279=ORIENTED_EDGE('',*,*,#8607,.F.);
#11280=ORIENTED_EDGE('',*,*,#8615,.T.);
#11281=ORIENTED_EDGE('',*,*,#8294,.F.);
#11282=ORIENTED_EDGE('',*,*,#8289,.F.);
#11283=ORIENTED_EDGE('',*,*,#8307,.T.);
#11284=ORIENTED_EDGE('',*,*,#8309,.T.);
#11285=ORIENTED_EDGE('',*,*,#8302,.F.);
#11286=ORIENTED_EDGE('',*,*,#8300,.T.);
#11287=ORIENTED_EDGE('',*,*,#8616,.T.);
#11288=ORIENTED_EDGE('',*,*,#8618,.F.);
#11289=ORIENTED_EDGE('',*,*,#8398,.F.);
#11290=ORIENTED_EDGE('',*,*,#8618,.T.);
#11291=ORIENTED_EDGE('',*,*,#8397,.F.);
#11292=ORIENTED_EDGE('',*,*,#8619,.T.);
#11293=ORIENTED_EDGE('',*,*,#8395,.F.);
#11294=ORIENTED_EDGE('',*,*,#8620,.F.);
#11295=ORIENTED_EDGE('',*,*,#8402,.F.);
#11296=ORIENTED_EDGE('',*,*,#8620,.T.);
#11297=ORIENTED_EDGE('',*,*,#8401,.F.);
#11298=ORIENTED_EDGE('',*,*,#8621,.T.);
#11299=ORIENTED_EDGE('',*,*,#8399,.F.);
#11300=ORIENTED_EDGE('',*,*,#8622,.F.);
#11301=ORIENTED_EDGE('',*,*,#8406,.F.);
#11302=ORIENTED_EDGE('',*,*,#8622,.T.);
#11303=ORIENTED_EDGE('',*,*,#8405,.F.);
#11304=ORIENTED_EDGE('',*,*,#8623,.T.);
#11305=ORIENTED_EDGE('',*,*,#8403,.F.);
#11306=ORIENTED_EDGE('',*,*,#8624,.F.);
#11307=ORIENTED_EDGE('',*,*,#8410,.F.);
#11308=ORIENTED_EDGE('',*,*,#8624,.T.);
#11309=ORIENTED_EDGE('',*,*,#8409,.F.);
#11310=ORIENTED_EDGE('',*,*,#8625,.T.);
#11311=ORIENTED_EDGE('',*,*,#8407,.F.);
#11312=ORIENTED_EDGE('',*,*,#8626,.F.);
#11313=ORIENTED_EDGE('',*,*,#8414,.F.);
#11314=ORIENTED_EDGE('',*,*,#8626,.T.);
#11315=ORIENTED_EDGE('',*,*,#8413,.F.);
#11316=ORIENTED_EDGE('',*,*,#8627,.T.);
#11317=ORIENTED_EDGE('',*,*,#8411,.F.);
#11318=ORIENTED_EDGE('',*,*,#8628,.F.);
#11319=ORIENTED_EDGE('',*,*,#8418,.F.);
#11320=ORIENTED_EDGE('',*,*,#8628,.T.);
#11321=ORIENTED_EDGE('',*,*,#8417,.F.);
#11322=ORIENTED_EDGE('',*,*,#8629,.T.);
#11323=ORIENTED_EDGE('',*,*,#8415,.F.);
#11324=ORIENTED_EDGE('',*,*,#8629,.F.);
#11325=ORIENTED_EDGE('',*,*,#8416,.F.);
#11326=ORIENTED_EDGE('',*,*,#8627,.F.);
#11327=ORIENTED_EDGE('',*,*,#8412,.F.);
#11328=ORIENTED_EDGE('',*,*,#8625,.F.);
#11329=ORIENTED_EDGE('',*,*,#8408,.F.);
#11330=ORIENTED_EDGE('',*,*,#8623,.F.);
#11331=ORIENTED_EDGE('',*,*,#8404,.F.);
#11332=ORIENTED_EDGE('',*,*,#8621,.F.);
#11333=ORIENTED_EDGE('',*,*,#8400,.F.);
#11334=ORIENTED_EDGE('',*,*,#8619,.F.);
#11335=ORIENTED_EDGE('',*,*,#8396,.F.);
#11336=ORIENTED_EDGE('',*,*,#8358,.F.);
#11337=ORIENTED_EDGE('',*,*,#8362,.F.);
#11338=ORIENTED_EDGE('',*,*,#8293,.F.);
#11339=ORIENTED_EDGE('',*,*,#8304,.F.);
#11340=ORIENTED_EDGE('',*,*,#8308,.F.);
#11341=ORIENTED_EDGE('',*,*,#8291,.F.);
#11342=ORIENTED_EDGE('',*,*,#8314,.F.);
#11343=ORIENTED_EDGE('',*,*,#8325,.F.);
#11344=ORIENTED_EDGE('',*,*,#8329,.F.);
#11345=ORIENTED_EDGE('',*,*,#8312,.F.);
#11346=ORIENTED_EDGE('',*,*,#8571,.F.);
#11347=ORIENTED_EDGE('',*,*,#8630,.F.);
#11348=ORIENTED_EDGE('',*,*,#8316,.F.);
#11349=ORIENTED_EDGE('',*,*,#8580,.F.);
#11350=ORIENTED_EDGE('',*,*,#8566,.F.);
#11351=ORIENTED_EDGE('',*,*,#8568,.F.);
#11352=ORIENTED_EDGE('',*,*,#8466,.F.);
#11353=ORIENTED_EDGE('',*,*,#8631,.T.);
#11354=ORIENTED_EDGE('',*,*,#8432,.F.);
#11355=ORIENTED_EDGE('',*,*,#8631,.F.);
#11356=ORIENTED_EDGE('',*,*,#8467,.F.);
#11357=ORIENTED_EDGE('',*,*,#8632,.T.);
#11358=ORIENTED_EDGE('',*,*,#8461,.F.);
#11359=ORIENTED_EDGE('',*,*,#8632,.F.);
#11360=ORIENTED_EDGE('',*,*,#8468,.F.);
#11361=ORIENTED_EDGE('',*,*,#8633,.T.);
#11362=ORIENTED_EDGE('',*,*,#8460,.F.);
#11363=ORIENTED_EDGE('',*,*,#8633,.F.);
#11364=ORIENTED_EDGE('',*,*,#8469,.F.);
#11365=ORIENTED_EDGE('',*,*,#8634,.T.);
#11366=ORIENTED_EDGE('',*,*,#8431,.F.);
#11367=ORIENTED_EDGE('',*,*,#8634,.F.);
#11368=ORIENTED_EDGE('',*,*,#8470,.F.);
#11369=ORIENTED_EDGE('',*,*,#8635,.T.);
#11370=ORIENTED_EDGE('',*,*,#8430,.F.);
#11371=ORIENTED_EDGE('',*,*,#8635,.F.);
#11372=ORIENTED_EDGE('',*,*,#8471,.F.);
#11373=ORIENTED_EDGE('',*,*,#8636,.T.);
#11374=ORIENTED_EDGE('',*,*,#8459,.F.);
#11375=ORIENTED_EDGE('',*,*,#8636,.F.);
#11376=ORIENTED_EDGE('',*,*,#8342,.F.);
#11377=ORIENTED_EDGE('',*,*,#8637,.T.);
#11378=ORIENTED_EDGE('',*,*,#8638,.T.);
#11379=ORIENTED_EDGE('',*,*,#8637,.F.);
#11380=ORIENTED_EDGE('',*,*,#8638,.F.);
#11381=ORIENTED_EDGE('',*,*,#8639,.T.);
#11382=ORIENTED_EDGE('',*,*,#8639,.F.);
#11383=ORIENTED_EDGE('',*,*,#8640,.T.);
#11384=ORIENTED_EDGE('',*,*,#8641,.T.);
#11385=ORIENTED_EDGE('',*,*,#8640,.F.);
#11386=ORIENTED_EDGE('',*,*,#8641,.F.);
#11387=ORIENTED_EDGE('',*,*,#8555,.T.);
#11388=ORIENTED_EDGE('',*,*,#8642,.T.);
#11389=ORIENTED_EDGE('',*,*,#8558,.F.);
#11390=ORIENTED_EDGE('',*,*,#8642,.F.);
#11391=ORIENTED_EDGE('',*,*,#8643,.T.);
#11392=ORIENTED_EDGE('',*,*,#8356,.F.);
#11393=ORIENTED_EDGE('',*,*,#8643,.F.);
#11394=ORIENTED_EDGE('',*,*,#8530,.F.);
#11395=ORIENTED_EDGE('',*,*,#8644,.T.);
#11396=ORIENTED_EDGE('',*,*,#8553,.T.);
#11397=ORIENTED_EDGE('',*,*,#8539,.F.);
#11398=ORIENTED_EDGE('',*,*,#8532,.F.);
#11399=ORIENTED_EDGE('',*,*,#8531,.F.);
#11400=ORIENTED_EDGE('',*,*,#8537,.F.);
#11401=ORIENTED_EDGE('',*,*,#8544,.F.);
#11402=ORIENTED_EDGE('',*,*,#8645,.T.);
#11403=ORIENTED_EDGE('',*,*,#8547,.F.);
#11404=ORIENTED_EDGE('',*,*,#8549,.T.);
#11405=ORIENTED_EDGE('',*,*,#8548,.F.);
#11406=ORIENTED_EDGE('',*,*,#8552,.F.);
#11407=ORIENTED_EDGE('',*,*,#8541,.F.);
#11408=ORIENTED_EDGE('',*,*,#8554,.T.);
#11409=ORIENTED_EDGE('',*,*,#8644,.F.);
#11410=ORIENTED_EDGE('',*,*,#8543,.F.);
#11411=ORIENTED_EDGE('',*,*,#8645,.F.);
#11412=ORIENTED_EDGE('',*,*,#8480,.F.);
#11413=ORIENTED_EDGE('',*,*,#8490,.T.);
#11414=ORIENTED_EDGE('',*,*,#8508,.F.);
#11415=ORIENTED_EDGE('',*,*,#8646,.F.);
#11416=ORIENTED_EDGE('',*,*,#8477,.F.);
#11417=ORIENTED_EDGE('',*,*,#8646,.T.);
#11418=ORIENTED_EDGE('',*,*,#8507,.F.);
#11419=ORIENTED_EDGE('',*,*,#8647,.F.);
#11420=ORIENTED_EDGE('',*,*,#8475,.F.);
#11421=ORIENTED_EDGE('',*,*,#8647,.T.);
#11422=ORIENTED_EDGE('',*,*,#8505,.F.);
#11423=ORIENTED_EDGE('',*,*,#8648,.F.);
#11424=ORIENTED_EDGE('',*,*,#8438,.F.);
#11425=ORIENTED_EDGE('',*,*,#8587,.F.);
#11426=ORIENTED_EDGE('',*,*,#8649,.T.);
#11427=ORIENTED_EDGE('',*,*,#8443,.F.);
#11428=ORIENTED_EDGE('',*,*,#8463,.F.);
#11429=ORIENTED_EDGE('',*,*,#8448,.T.);
#11430=ORIENTED_EDGE('',*,*,#8613,.F.);
#11431=ORIENTED_EDGE('',*,*,#8650,.F.);
#11432=ORIENTED_EDGE('',*,*,#8585,.F.);
#11433=ORIENTED_EDGE('',*,*,#8650,.T.);
#11434=ORIENTED_EDGE('',*,*,#8609,.F.);
#11435=ORIENTED_EDGE('',*,*,#8600,.F.);
#11436=ORIENTED_EDGE('',*,*,#8614,.T.);
#11437=ORIENTED_EDGE('',*,*,#8456,.F.);
#11438=ORIENTED_EDGE('',*,*,#8368,.F.);
#11439=ORIENTED_EDGE('',*,*,#8296,.F.);
#11440=ORIENTED_EDGE('',*,*,#8589,.F.);
#11441=ORIENTED_EDGE('',*,*,#8576,.T.);
#11442=ORIENTED_EDGE('',*,*,#8444,.F.);
#11443=ORIENTED_EDGE('',*,*,#8649,.F.);
#11444=ORIENTED_EDGE('',*,*,#8503,.F.);
#11445=ORIENTED_EDGE('',*,*,#8511,.F.);
#11446=ORIENTED_EDGE('',*,*,#8439,.F.);
#11447=ORIENTED_EDGE('',*,*,#8648,.T.);
#11448=ORIENTED_EDGE('',*,*,#8579,.T.);
#11449=ORIENTED_EDGE('',*,*,#8319,.T.);
#11450=ORIENTED_EDGE('',*,*,#8382,.F.);
#11451=ORIENTED_EDGE('',*,*,#8426,.F.);
#11452=ORIENTED_EDGE('',*,*,#8491,.T.);
#11453=ORIENTED_EDGE('',*,*,#8427,.F.);
#11454=ORIENTED_EDGE('',*,*,#8380,.F.);
#11455=ORIENTED_EDGE('',*,*,#8651,.T.);
#11456=ORIENTED_EDGE('',*,*,#8617,.T.);
#11457=ORIENTED_EDGE('',*,*,#8298,.T.);
#11458=ORIENTED_EDGE('',*,*,#8367,.F.);
#11459=ORIENTED_EDGE('',*,*,#8363,.F.);
#11460=ORIENTED_EDGE('',*,*,#8391,.F.);
#11461=ORIENTED_EDGE('',*,*,#8598,.F.);
#11462=ORIENTED_EDGE('',*,*,#8604,.F.);
#11463=ORIENTED_EDGE('',*,*,#8630,.T.);
#11464=ORIENTED_EDGE('',*,*,#8570,.F.);
#11465=ORIENTED_EDGE('',*,*,#8599,.T.);
#11466=ORIENTED_EDGE('',*,*,#8389,.F.);
#11467=ORIENTED_EDGE('',*,*,#8375,.F.);
#11468=ORIENTED_EDGE('',*,*,#8383,.F.);
#11469=ORIENTED_EDGE('',*,*,#8317,.F.);
#11470=ORIENTED_EDGE('',*,*,#8492,.T.);
#11471=ORIENTED_EDGE('',*,*,#8651,.F.);
#11472=ORIENTED_EDGE('',*,*,#8379,.F.);
#11473=ORIENTED_EDGE('',*,*,#8652,.T.);
#11474=ORIENTED_EDGE('',*,*,#8525,.T.);
#11475=ORIENTED_EDGE('',*,*,#8653,.F.);
#11476=ORIENTED_EDGE('',*,*,#8370,.F.);
#11477=ORIENTED_EDGE('',*,*,#8455,.F.);
#11478=ORIENTED_EDGE('',*,*,#8524,.T.);
#11479=ORIENTED_EDGE('',*,*,#8654,.F.);
#11480=ORIENTED_EDGE('',*,*,#8371,.F.);
#11481=ORIENTED_EDGE('',*,*,#8653,.T.);
#11482=ORIENTED_EDGE('',*,*,#8523,.T.);
#11483=ORIENTED_EDGE('',*,*,#8516,.F.);
#11484=ORIENTED_EDGE('',*,*,#8486,.F.);
#11485=ORIENTED_EDGE('',*,*,#8392,.F.);
#11486=ORIENTED_EDGE('',*,*,#8365,.F.);
#11487=ORIENTED_EDGE('',*,*,#8372,.F.);
#11488=ORIENTED_EDGE('',*,*,#8654,.T.);
#11489=ORIENTED_EDGE('',*,*,#8493,.T.);
#11490=ORIENTED_EDGE('',*,*,#8652,.F.);
#11491=ORIENTED_EDGE('',*,*,#8378,.F.);
#11492=ORIENTED_EDGE('',*,*,#8373,.F.);
#11493=ORIENTED_EDGE('',*,*,#8394,.F.);
#11494=ORIENTED_EDGE('',*,*,#8485,.T.);
#11495=ORIENTED_EDGE('',*,*,#8482,.F.);
#15714=PLANE('',#17192);
#15715=PLANE('',#17193);
#15716=PLANE('',#17194);
#15717=PLANE('',#17200);
#15718=PLANE('',#17201);
#15719=PLANE('',#17202);
#15720=PLANE('',#17210);
#15721=PLANE('',#17221);
#15722=PLANE('',#17253);
#15723=PLANE('',#17257);
#15724=PLANE('',#17272);
#15725=PLANE('',#17280);
#15726=PLANE('',#17299);
#15727=PLANE('',#17300);
#15728=PLANE('',#17325);
#15729=PLANE('',#17337);
#15730=PLANE('',#17348);
#15731=PLANE('',#17365);
#15732=PLANE('',#17368);
#15733=PLANE('',#17393);
#15734=PLANE('',#17406);
#15735=PLANE('',#17409);
#15736=PLANE('',#17413);
#15737=PLANE('',#17417);
#15738=PLANE('',#17421);
#15739=PLANE('',#17425);
#15740=PLANE('',#17429);
#15741=PLANE('',#17433);
#15742=PLANE('',#17437);
#15743=PLANE('',#17438);
#15744=PLANE('',#17439);
#15745=PLANE('',#17440);
#15746=PLANE('',#17441);
#15747=PLANE('',#17442);
#15748=PLANE('',#17443);
#15749=PLANE('',#17444);
#15750=PLANE('',#17445);
#15751=PLANE('',#17446);
#15752=PLANE('',#17447);
#15753=PLANE('',#17457);
#15754=PLANE('',#17461);
#15755=PLANE('',#17462);
#15756=PLANE('',#17467);
#15757=PLANE('',#17469);
#15758=PLANE('',#17472);
#15759=PLANE('',#17474);
#15760=PLANE('',#17475);
#15761=PLANE('',#17480);
#15762=PLANE('',#17482);
#15976=ADVANCED_FACE('',(#1805),#15714,.T.);
#15977=ADVANCED_FACE('',(#1806),#15715,.T.);
#15978=ADVANCED_FACE('',(#1807),#15716,.T.);
#15979=ADVANCED_FACE('',(#1808),#1226,.F.);
#15980=ADVANCED_FACE('',(#1809),#15717,.T.);
#15981=ADVANCED_FACE('',(#1810),#15718,.T.);
#15982=ADVANCED_FACE('',(#1811),#15719,.T.);
#15983=ADVANCED_FACE('',(#1812),#1227,.F.);
#15984=ADVANCED_FACE('',(#1813),#564,.F.);
#15985=ADVANCED_FACE('',(#1814,#414,#415,#416),#15720,.F.);
#15986=ADVANCED_FACE('',(#1815),#565,.F.);
#15987=ADVANCED_FACE('',(#1816),#566,.F.);
#15988=ADVANCED_FACE('',(#1817,#417,#418,#419),#15721,.T.);
#15989=ADVANCED_FACE('',(#1818),#1228,.F.);
#15990=ADVANCED_FACE('',(#1819),#567,.F.);
#15991=ADVANCED_FACE('',(#1820),#1229,.F.);
#15992=ADVANCED_FACE('',(#1821),#367,.T.);
#15993=ADVANCED_FACE('',(#1822),#568,.T.);
#15994=ADVANCED_FACE('',(#1823),#368,.T.);
#15995=ADVANCED_FACE('',(#1824),#569,.T.);
#15996=ADVANCED_FACE('',(#1825),#369,.T.);
#15997=ADVANCED_FACE('',(#1826),#570,.T.);
#15998=ADVANCED_FACE('',(#1827,#420,#421,#422,#423,#424,#425),#15722,.T.);
#15999=ADVANCED_FACE('',(#1828),#370,.T.);
#16000=ADVANCED_FACE('',(#1829,#426,#427,#428),#15723,.T.);
#16001=ADVANCED_FACE('',(#1830),#371,.T.);
#16002=ADVANCED_FACE('',(#1831),#1230,.T.);
#16003=ADVANCED_FACE('',(#1832),#372,.T.);
#16004=ADVANCED_FACE('',(#1833,#429,#430,#431),#15724,.T.);
#16005=ADVANCED_FACE('',(#1834),#373,.T.);
#16006=ADVANCED_FACE('',(#1835),#374,.T.);
#16007=ADVANCED_FACE('',(#1836,#432,#433,#434,#435,#436,#437,#438),#15725,
 .T.);
#16008=ADVANCED_FACE('',(#1837),#375,.T.);
#16009=ADVANCED_FACE('',(#1838),#1231,.T.);
#16010=ADVANCED_FACE('',(#1839),#376,.T.);
#16011=ADVANCED_FACE('',(#1840),#1232,.T.);
#16012=ADVANCED_FACE('',(#1841),#15726,.T.);
#16013=ADVANCED_FACE('',(#1842),#15727,.F.);
#16014=ADVANCED_FACE('',(#1843),#1233,.T.);
#16015=ADVANCED_FACE('',(#1844),#377,.T.);
#16016=ADVANCED_FACE('',(#1845),#1234,.T.);
#16017=ADVANCED_FACE('',(#1846),#378,.T.);
#16018=ADVANCED_FACE('',(#1847),#1235,.T.);
#16019=ADVANCED_FACE('',(#1848),#379,.T.);
#16020=ADVANCED_FACE('',(#1849),#1236,.T.);
#16021=ADVANCED_FACE('',(#1850),#380,.T.);
#16022=ADVANCED_FACE('',(#1851),#1237,.T.);
#16023=ADVANCED_FACE('',(#1852),#15728,.T.);
#16024=ADVANCED_FACE('',(#1853),#1238,.T.);
#16025=ADVANCED_FACE('',(#1854),#1239,.T.);
#16026=ADVANCED_FACE('',(#1855),#1240,.T.);
#16027=ADVANCED_FACE('',(#1856),#381,.T.);
#16028=ADVANCED_FACE('',(#1857),#382,.T.);
#16029=ADVANCED_FACE('',(#1858),#15729,.F.);
#16030=ADVANCED_FACE('',(#1859),#383,.T.);
#16031=ADVANCED_FACE('',(#1860),#571,.F.);
#16032=ADVANCED_FACE('',(#1861),#337,.F.);
#16033=ADVANCED_FACE('',(#1862),#1241,.T.);
#16034=ADVANCED_FACE('',(#1863),#1242,.T.);
#16035=ADVANCED_FACE('',(#1864),#338,.F.);
#16036=ADVANCED_FACE('',(#1865),#15730,.F.);
#16037=ADVANCED_FACE('',(#1866),#1243,.F.);
#16038=ADVANCED_FACE('',(#1867),#384,.T.);
#16039=ADVANCED_FACE('',(#1868),#1244,.T.);
#16040=ADVANCED_FACE('',(#1869),#385,.T.);
#16041=ADVANCED_FACE('',(#1870),#1245,.T.);
#16042=ADVANCED_FACE('',(#1871),#15731,.T.);
#16043=ADVANCED_FACE('',(#1872),#1246,.T.);
#16044=ADVANCED_FACE('',(#1873),#15732,.T.);
#16045=ADVANCED_FACE('',(#1874),#386,.T.);
#16046=ADVANCED_FACE('',(#1875),#387,.T.);
#16047=ADVANCED_FACE('',(#1876),#1247,.T.);
#16048=ADVANCED_FACE('',(#1877),#388,.T.);
#16049=ADVANCED_FACE('',(#1878),#1248,.T.);
#16050=ADVANCED_FACE('',(#1879),#389,.T.);
#16051=ADVANCED_FACE('',(#1880),#1249,.T.);
#16052=ADVANCED_FACE('',(#1881),#390,.T.);
#16053=ADVANCED_FACE('',(#1882),#1250,.T.);
#16054=ADVANCED_FACE('',(#1883),#1251,.T.);
#16055=ADVANCED_FACE('',(#1884),#15733,.T.);
#16056=ADVANCED_FACE('',(#1885),#1252,.T.);
#16057=ADVANCED_FACE('',(#1886),#1253,.T.);
#16058=ADVANCED_FACE('',(#1887),#391,.T.);
#16059=ADVANCED_FACE('',(#1888),#1254,.T.);
#16060=ADVANCED_FACE('',(#1889),#392,.T.);
#16061=ADVANCED_FACE('',(#1890),#15734,.T.);
#16062=ADVANCED_FACE('',(#1891),#15735,.T.);
#16063=ADVANCED_FACE('',(#1892),#393,.T.);
#16064=ADVANCED_FACE('',(#1893),#15736,.T.);
#16065=ADVANCED_FACE('',(#1894),#1255,.T.);
#16066=ADVANCED_FACE('',(#1895),#15737,.T.);
#16067=ADVANCED_FACE('',(#1896),#1256,.T.);
#16068=ADVANCED_FACE('',(#1897),#15738,.T.);
#16069=ADVANCED_FACE('',(#1898),#1257,.T.);
#16070=ADVANCED_FACE('',(#1899),#15739,.T.);
#16071=ADVANCED_FACE('',(#1900),#1258,.T.);
#16072=ADVANCED_FACE('',(#1901),#15740,.T.);
#16073=ADVANCED_FACE('',(#1902),#1259,.T.);
#16074=ADVANCED_FACE('',(#1903),#15741,.T.);
#16075=ADVANCED_FACE('',(#1904),#1260,.T.);
#16076=ADVANCED_FACE('',(#1905),#15742,.T.);
#16077=ADVANCED_FACE('',(#1906),#15743,.T.);
#16078=ADVANCED_FACE('',(#1907),#15744,.T.);
#16079=ADVANCED_FACE('',(#1908),#15745,.T.);
#16080=ADVANCED_FACE('',(#1909),#15746,.T.);
#16081=ADVANCED_FACE('',(#1910),#15747,.T.);
#16082=ADVANCED_FACE('',(#1911),#15748,.T.);
#16083=ADVANCED_FACE('',(#1912),#15749,.T.);
#16084=ADVANCED_FACE('',(#1913),#15750,.F.);
#16085=ADVANCED_FACE('',(#1914),#15751,.F.);
#16086=ADVANCED_FACE('',(#1915),#15752,.T.);
#16087=ADVANCED_FACE('',(#1916),#1261,.F.);
#16088=ADVANCED_FACE('',(#1917),#1262,.F.);
#16089=ADVANCED_FACE('',(#1918),#1263,.F.);
#16090=ADVANCED_FACE('',(#1919),#1264,.F.);
#16091=ADVANCED_FACE('',(#1920),#1265,.F.);
#16092=ADVANCED_FACE('',(#1921),#1266,.F.);
#16093=ADVANCED_FACE('',(#1922),#1267,.F.);
#16094=ADVANCED_FACE('',(#1923,#439),#15753,.F.);
#16095=ADVANCED_FACE('',(#1924),#1268,.F.);
#16096=ADVANCED_FACE('',(#1925,#440),#15754,.F.);
#16097=ADVANCED_FACE('',(#1926,#441),#15755,.F.);
#16098=ADVANCED_FACE('',(#1927),#1269,.F.);
#16099=ADVANCED_FACE('',(#1928),#572,.F.);
#16100=ADVANCED_FACE('',(#1929),#15756,.F.);
#16101=ADVANCED_FACE('',(#1930),#1270,.T.);
#16102=ADVANCED_FACE('',(#1931),#15757,.T.);
#16103=ADVANCED_FACE('',(#1932),#1271,.T.);
#16104=ADVANCED_FACE('',(#1933),#1272,.T.);
#16105=ADVANCED_FACE('',(#1934),#15758,.T.);
#16106=ADVANCED_FACE('',(#1935),#1273,.T.);
#16107=ADVANCED_FACE('',(#1936),#15759,.T.);
#16108=ADVANCED_FACE('',(#1937),#15760,.T.);
#16109=ADVANCED_FACE('',(#1938),#1274,.T.);
#16110=ADVANCED_FACE('',(#1939),#1275,.T.);
#16111=ADVANCED_FACE('',(#1940),#1276,.T.);
#16112=ADVANCED_FACE('',(#1941),#1277,.T.);
#16113=ADVANCED_FACE('',(#1942),#15761,.T.);
#16114=ADVANCED_FACE('',(#1943),#1278,.T.);
#16115=ADVANCED_FACE('',(#1944),#15762,.T.);
#16116=ADVANCED_FACE('',(#1945),#1279,.T.);
#16117=ADVANCED_FACE('',(#1946),#1280,.T.);
#16949=CLOSED_SHELL('',(#15976,#15977,#15978,#15979,#15980,#15981,#15982,
#15983,#15984,#15985,#15986,#15987,#15988,#15989,#15990,#15991,#15992,#15993,
#15994,#15995,#15996,#15997,#15998,#15999,#16000,#16001,#16002,#16003,#16004,
#16005,#16006,#16007,#16008,#16009,#16010,#16011,#16012,#16013,#16014,#16015,
#16016,#16017,#16018,#16019,#16020,#16021,#16022,#16023,#16024,#16025,#16026,
#16027,#16028,#16029,#16030,#16031,#16032,#16033,#16034,#16035,#16036,#16037,
#16038,#16039,#16040,#16041,#16042,#16043,#16044,#16045,#16046,#16047,#16048,
#16049,#16050,#16051,#16052,#16053,#16054,#16055,#16056,#16057,#16058,#16059,
#16060,#16061,#16062,#16063,#16064,#16065,#16066,#16067,#16068,#16069,#16070,
#16071,#16072,#16073,#16074,#16075,#16076,#16077,#16078,#16079,#16080,#16081,
#16082,#16083,#16084,#16085,#16086,#16087,#16088,#16089,#16090,#16091,#16092,
#16093,#16094,#16095,#16096,#16097,#16098,#16099,#16100,#16101,#16102,#16103,
#16104,#16105,#16106,#16107,#16108,#16109,#16110,#16111,#16112,#16113,#16114,
#16115,#16116,#16117));
#17191=AXIS2_PLACEMENT_3D('',#22942,#18791,#18792);
#17192=AXIS2_PLACEMENT_3D('',#22943,#18793,#18794);
#17193=AXIS2_PLACEMENT_3D('',#22959,#18798,#18799);
#17194=AXIS2_PLACEMENT_3D('',#22993,#18806,#18807);
#17195=AXIS2_PLACEMENT_3D('',#23006,#18810,#18811);
#17196=AXIS2_PLACEMENT_3D('',#23008,#18812,#18813);
#17197=AXIS2_PLACEMENT_3D('',#23011,#18815,#18816);
#17198=AXIS2_PLACEMENT_3D('',#23012,#18817,#18818);
#17199=AXIS2_PLACEMENT_3D('',#23013,#18819,#18820);
#17200=AXIS2_PLACEMENT_3D('',#23014,#18821,#18822);
#17201=AXIS2_PLACEMENT_3D('',#23030,#18826,#18827);
#17202=AXIS2_PLACEMENT_3D('',#23064,#18834,#18835);
#17203=AXIS2_PLACEMENT_3D('',#23077,#18838,#18839);
#17204=AXIS2_PLACEMENT_3D('',#23079,#18840,#18841);
#17205=AXIS2_PLACEMENT_3D('',#23082,#18843,#18844);
#17206=AXIS2_PLACEMENT_3D('',#23083,#18845,#18846);
#17207=AXIS2_PLACEMENT_3D('',#23084,#18847,#18848);
#17208=AXIS2_PLACEMENT_3D('',#23085,#18849,#18850);
#17209=AXIS2_PLACEMENT_3D('',#23087,#18851,#18852);
#17210=AXIS2_PLACEMENT_3D('',#23089,#18854,#18855);
#17211=AXIS2_PLACEMENT_3D('',#23092,#18856,#18857);
#17212=AXIS2_PLACEMENT_3D('',#23096,#18859,#18860);
#17213=AXIS2_PLACEMENT_3D('',#23100,#18862,#18863);
#17214=AXIS2_PLACEMENT_3D('',#23104,#18865,#18866);
#17215=AXIS2_PLACEMENT_3D('',#23107,#18868,#18869);
#17216=AXIS2_PLACEMENT_3D('',#23109,#18870,#18871);
#17217=AXIS2_PLACEMENT_3D('',#23110,#18872,#18873);
#17218=AXIS2_PLACEMENT_3D('',#23112,#18875,#18876);
#17219=AXIS2_PLACEMENT_3D('',#23114,#18877,#18878);
#17220=AXIS2_PLACEMENT_3D('',#23117,#18880,#18881);
#17221=AXIS2_PLACEMENT_3D('',#23118,#18882,#18883);
#17222=AXIS2_PLACEMENT_3D('',#23123,#18885,#18886);
#17223=AXIS2_PLACEMENT_3D('',#23127,#18888,#18889);
#17224=AXIS2_PLACEMENT_3D('',#23131,#18891,#18892);
#17225=AXIS2_PLACEMENT_3D('',#23134,#18894,#18895);
#17226=AXIS2_PLACEMENT_3D('',#23136,#18896,#18897);
#17227=AXIS2_PLACEMENT_3D('',#23138,#18898,#18899);
#17228=AXIS2_PLACEMENT_3D('',#23139,#18900,#18901);
#17229=AXIS2_PLACEMENT_3D('',#23142,#18903,#18904);
#17230=AXIS2_PLACEMENT_3D('',#23143,#18905,#18906);
#17231=AXIS2_PLACEMENT_3D('',#23146,#18908,#18909);
#17232=AXIS2_PLACEMENT_3D('',#23147,#18910,#18911);
#17233=AXIS2_PLACEMENT_3D('',#23150,#18913,#18914);
#17234=AXIS2_PLACEMENT_3D('',#23151,#18915,#18916);
#17235=AXIS2_PLACEMENT_3D('',#23163,#18917,#18918);
#17236=AXIS2_PLACEMENT_3D('',#23173,#18919,#18920);
#17237=AXIS2_PLACEMENT_3D('',#23174,#18921,#18922);
#17238=AXIS2_PLACEMENT_3D('',#23187,#18923,#18924);
#17239=AXIS2_PLACEMENT_3D('',#23203,#18925,#18926);
#17240=AXIS2_PLACEMENT_3D('',#23215,#18927,#18928);
#17241=AXIS2_PLACEMENT_3D('',#23226,#18929,#18930);
#17242=AXIS2_PLACEMENT_3D('',#23227,#18931,#18932);
#17243=AXIS2_PLACEMENT_3D('',#23228,#18933,#18934);
#17244=AXIS2_PLACEMENT_3D('',#23246,#18935,#18936);
#17245=AXIS2_PLACEMENT_3D('',#23257,#18937,#18938);
#17246=AXIS2_PLACEMENT_3D('',#23259,#18939,#18940);
#17247=AXIS2_PLACEMENT_3D('',#23261,#18941,#18942);
#17248=AXIS2_PLACEMENT_3D('',#23263,#18943,#18944);
#17249=AXIS2_PLACEMENT_3D('',#23264,#18945,#18946);
#17250=AXIS2_PLACEMENT_3D('',#23265,#18947,#18948);
#17251=AXIS2_PLACEMENT_3D('',#23284,#18950,#18951);
#17252=AXIS2_PLACEMENT_3D('',#23315,#18952,#18953);
#17253=AXIS2_PLACEMENT_3D('',#23331,#18954,#18955);
#17254=AXIS2_PLACEMENT_3D('',#23380,#18980,#18981);
#17255=AXIS2_PLACEMENT_3D('',#23394,#18982,#18983);
#17256=AXIS2_PLACEMENT_3D('',#23411,#18984,#18985);
#17257=AXIS2_PLACEMENT_3D('',#23412,#18986,#18987);
#17258=AXIS2_PLACEMENT_3D('',#23434,#18992,#18993);
#17259=AXIS2_PLACEMENT_3D('',#23436,#18994,#18995);
#17260=AXIS2_PLACEMENT_3D('',#23438,#18996,#18997);
#17261=AXIS2_PLACEMENT_3D('',#23439,#18998,#18999);
#17262=AXIS2_PLACEMENT_3D('',#23450,#19000,#19001);
#17263=AXIS2_PLACEMENT_3D('',#23452,#19002,#19003);
#17264=AXIS2_PLACEMENT_3D('',#23459,#19004,#19005);
#17265=AXIS2_PLACEMENT_3D('',#23473,#19006,#19007);
#17266=AXIS2_PLACEMENT_3D('',#23487,#19008,#19009);
#17267=AXIS2_PLACEMENT_3D('',#23496,#19010,#19011);
#17268=AXIS2_PLACEMENT_3D('',#23505,#19013,#19014);
#17269=AXIS2_PLACEMENT_3D('',#23506,#19015,#19016);
#17270=AXIS2_PLACEMENT_3D('',#23514,#19017,#19018);
#17271=AXIS2_PLACEMENT_3D('',#23527,#19019,#19020);
#17272=AXIS2_PLACEMENT_3D('',#23536,#19021,#19022);
#17273=AXIS2_PLACEMENT_3D('',#23558,#19027,#19028);
#17274=AXIS2_PLACEMENT_3D('',#23560,#19029,#19030);
#17275=AXIS2_PLACEMENT_3D('',#23562,#19031,#19032);
#17276=AXIS2_PLACEMENT_3D('',#23563,#19033,#19034);
#17277=AXIS2_PLACEMENT_3D('',#23580,#19035,#19036);
#17278=AXIS2_PLACEMENT_3D('',#23582,#19037,#19038);
#17279=AXIS2_PLACEMENT_3D('',#23583,#19039,#19040);
#17280=AXIS2_PLACEMENT_3D('',#23584,#19041,#19042);
#17281=AXIS2_PLACEMENT_3D('',#23586,#19043,#19044);
#17282=AXIS2_PLACEMENT_3D('',#23588,#19045,#19046);
#17283=AXIS2_PLACEMENT_3D('',#23590,#19047,#19048);
#17284=AXIS2_PLACEMENT_3D('',#23592,#19049,#19050);
#17285=AXIS2_PLACEMENT_3D('',#23594,#19051,#19052);
#17286=AXIS2_PLACEMENT_3D('',#23596,#19053,#19054);
#17287=AXIS2_PLACEMENT_3D('',#23598,#19055,#19056);
#17288=AXIS2_PLACEMENT_3D('',#23599,#19057,#19058);
#17289=AXIS2_PLACEMENT_3D('',#23601,#19059,#19060);
#17290=AXIS2_PLACEMENT_3D('',#23603,#19061,#19062);
#17291=AXIS2_PLACEMENT_3D('',#23604,#19063,#19064);
#17292=AXIS2_PLACEMENT_3D('',#23605,#19065,#19066);
#17293=AXIS2_PLACEMENT_3D('',#23608,#19067,#19068);
#17294=AXIS2_PLACEMENT_3D('',#23611,#19071,#19072);
#17295=AXIS2_PLACEMENT_3D('',#23614,#19073,#19074);
#17296=AXIS2_PLACEMENT_3D('',#23615,#19075,#19076);
#17297=AXIS2_PLACEMENT_3D('',#23616,#19077,#19078);
#17298=AXIS2_PLACEMENT_3D('',#23617,#19079,#19080);
#17299=AXIS2_PLACEMENT_3D('',#23628,#19083,#19084);
#17300=AXIS2_PLACEMENT_3D('',#23639,#19091,#19092);
#17301=AXIS2_PLACEMENT_3D('',#23641,#19093,#19094);
#17302=AXIS2_PLACEMENT_3D('',#23644,#19096,#19097);
#17303=AXIS2_PLACEMENT_3D('',#23645,#19098,#19099);
#17304=AXIS2_PLACEMENT_3D('',#23646,#19100,#19101);
#17305=AXIS2_PLACEMENT_3D('',#23647,#19102,#19103);
#17306=AXIS2_PLACEMENT_3D('',#23648,#19104,#19105);
#17307=AXIS2_PLACEMENT_3D('',#23650,#19106,#19107);
#17308=AXIS2_PLACEMENT_3D('',#23651,#19108,#19109);
#17309=AXIS2_PLACEMENT_3D('',#23652,#19110,#19111);
#17310=AXIS2_PLACEMENT_3D('',#23654,#19112,#19113);
#17311=AXIS2_PLACEMENT_3D('',#23656,#19115,#19116);
#17312=AXIS2_PLACEMENT_3D('',#23658,#19117,#19118);
#17313=AXIS2_PLACEMENT_3D('',#23659,#19119,#19120);
#17314=AXIS2_PLACEMENT_3D('',#23660,#19121,#19122);
#17315=AXIS2_PLACEMENT_3D('',#23662,#19123,#19124);
#17316=AXIS2_PLACEMENT_3D('',#23664,#19126,#19127);
#17317=AXIS2_PLACEMENT_3D('',#23666,#19128,#19129);
#17318=AXIS2_PLACEMENT_3D('',#23667,#19130,#19131);
#17319=AXIS2_PLACEMENT_3D('',#23668,#19132,#19133);
#17320=AXIS2_PLACEMENT_3D('',#23670,#19134,#19135);
#17321=AXIS2_PLACEMENT_3D('',#23672,#19137,#19138);
#17322=AXIS2_PLACEMENT_3D('',#23673,#19139,#19140);
#17323=AXIS2_PLACEMENT_3D('',#23674,#19141,#19142);
#17324=AXIS2_PLACEMENT_3D('',#23677,#19144,#19145);
#17325=AXIS2_PLACEMENT_3D('',#23679,#19147,#19148);
#17326=AXIS2_PLACEMENT_3D('',#23683,#19151,#19152);
#17327=AXIS2_PLACEMENT_3D('',#23684,#19153,#19154);
#17328=AXIS2_PLACEMENT_3D('',#23685,#19155,#19156);
#17329=AXIS2_PLACEMENT_3D('',#23687,#19157,#19158);
#17330=AXIS2_PLACEMENT_3D('',#23696,#19160,#19161);
#17331=AXIS2_PLACEMENT_3D('',#23698,#19162,#19163);
#17332=AXIS2_PLACEMENT_3D('',#23701,#19165,#19166);
#17333=AXIS2_PLACEMENT_3D('',#23702,#19167,#19168);
#17334=AXIS2_PLACEMENT_3D('',#23703,#19169,#19170);
#17335=AXIS2_PLACEMENT_3D('',#23704,#19171,#19172);
#17336=AXIS2_PLACEMENT_3D('',#23705,#19173,#19174);
#17337=AXIS2_PLACEMENT_3D('',#23706,#19175,#19176);
#17338=AXIS2_PLACEMENT_3D('',#23708,#19177,#19178);
#17339=AXIS2_PLACEMENT_3D('',#23711,#19180,#19181);
#17340=AXIS2_PLACEMENT_3D('',#23712,#19182,#19183);
#17341=AXIS2_PLACEMENT_3D('',#23714,#19184,#19185);
#17342=AXIS2_PLACEMENT_3D('',#23716,#19186,#19187);
#17343=AXIS2_PLACEMENT_3D('',#23717,#19188,#19189);
#17344=AXIS2_PLACEMENT_3D('',#23718,#19190,#19191);
#17345=AXIS2_PLACEMENT_3D('',#23721,#19193,#19194);
#17346=AXIS2_PLACEMENT_3D('',#24051,#19195,#19196);
#17347=AXIS2_PLACEMENT_3D('',#24109,#19199,#19200);
#17348=AXIS2_PLACEMENT_3D('',#24408,#19203,#19204);
#17349=AXIS2_PLACEMENT_3D('',#24410,#19205,#19206);
#17350=AXIS2_PLACEMENT_3D('',#24411,#19207,#19208);
#17351=AXIS2_PLACEMENT_3D('',#24412,#19209,#19210);
#17352=AXIS2_PLACEMENT_3D('',#24414,#19211,#19212);
#17353=AXIS2_PLACEMENT_3D('',#24418,#19215,#19216);
#17354=AXIS2_PLACEMENT_3D('',#24419,#19217,#19218);
#17355=AXIS2_PLACEMENT_3D('',#24421,#19219,#19220);
#17356=AXIS2_PLACEMENT_3D('',#24423,#19221,#19222);
#17357=AXIS2_PLACEMENT_3D('',#24424,#19223,#19224);
#17358=AXIS2_PLACEMENT_3D('',#24425,#19225,#19226);
#17359=AXIS2_PLACEMENT_3D('',#24442,#19229,#19230);
#17360=AXIS2_PLACEMENT_3D('',#24444,#19232,#19233);
#17361=AXIS2_PLACEMENT_3D('',#24447,#19234,#19235);
#17362=AXIS2_PLACEMENT_3D('',#24448,#19236,#19237);
#17363=AXIS2_PLACEMENT_3D('',#24449,#19238,#19239);
#17364=AXIS2_PLACEMENT_3D('',#24450,#19240,#19241);
#17365=AXIS2_PLACEMENT_3D('',#24461,#19244,#19245);
#17366=AXIS2_PLACEMENT_3D('',#24467,#19249,#19250);
#17367=AXIS2_PLACEMENT_3D('',#24470,#19252,#19253);
#17368=AXIS2_PLACEMENT_3D('',#24471,#19254,#19255);
#17369=AXIS2_PLACEMENT_3D('',#24472,#19256,#19257);
#17370=AXIS2_PLACEMENT_3D('',#24473,#19258,#19259);
#17371=AXIS2_PLACEMENT_3D('',#24474,#19260,#19261);
#17372=AXIS2_PLACEMENT_3D('',#24475,#19262,#19263);
#17373=AXIS2_PLACEMENT_3D('',#24476,#19264,#19265);
#17374=AXIS2_PLACEMENT_3D('',#24478,#19266,#19267);
#17375=AXIS2_PLACEMENT_3D('',#24480,#19268,#19269);
#17376=AXIS2_PLACEMENT_3D('',#24481,#19270,#19271);
#17377=AXIS2_PLACEMENT_3D('',#24482,#19272,#19273);
#17378=AXIS2_PLACEMENT_3D('',#24484,#19274,#19275);
#17379=AXIS2_PLACEMENT_3D('',#24486,#19277,#19278);
#17380=AXIS2_PLACEMENT_3D('',#24488,#19279,#19280);
#17381=AXIS2_PLACEMENT_3D('',#24489,#19281,#19282);
#17382=AXIS2_PLACEMENT_3D('',#24490,#19283,#19284);
#17383=AXIS2_PLACEMENT_3D('',#24491,#19285,#19286);
#17384=AXIS2_PLACEMENT_3D('',#24493,#19288,#19289);
#17385=AXIS2_PLACEMENT_3D('',#24494,#19290,#19291);
#17386=AXIS2_PLACEMENT_3D('',#24495,#19292,#19293);
#17387=AXIS2_PLACEMENT_3D('',#24496,#19294,#19295);
#17388=AXIS2_PLACEMENT_3D('',#24497,#19296,#19297);
#17389=AXIS2_PLACEMENT_3D('',#24499,#19298,#19299);
#17390=AXIS2_PLACEMENT_3D('',#24500,#19300,#19301);
#17391=AXIS2_PLACEMENT_3D('',#24501,#19302,#19303);
#17392=AXIS2_PLACEMENT_3D('',#24503,#19305,#19306);
#17393=AXIS2_PLACEMENT_3D('',#24505,#19308,#19309);
#17394=AXIS2_PLACEMENT_3D('',#24512,#19314,#19315);
#17395=AXIS2_PLACEMENT_3D('',#24515,#19317,#19318);
#17396=AXIS2_PLACEMENT_3D('',#24516,#19319,#19320);
#17397=AXIS2_PLACEMENT_3D('',#24518,#19321,#19322);
#17398=AXIS2_PLACEMENT_3D('',#24527,#19324,#19325);
#17399=AXIS2_PLACEMENT_3D('',#24529,#19326,#19327);
#17400=AXIS2_PLACEMENT_3D('',#24530,#19328,#19329);
#17401=AXIS2_PLACEMENT_3D('',#24531,#19330,#19331);
#17402=AXIS2_PLACEMENT_3D('',#24548,#19334,#19335);
#17403=AXIS2_PLACEMENT_3D('',#24550,#19337,#19338);
#17404=AXIS2_PLACEMENT_3D('',#24551,#19339,#19340);
#17405=AXIS2_PLACEMENT_3D('',#24552,#19341,#19342);
#17406=AXIS2_PLACEMENT_3D('',#24553,#19343,#19344);
#17407=AXIS2_PLACEMENT_3D('',#24554,#19345,#19346);
#17408=AXIS2_PLACEMENT_3D('',#24555,#19347,#19348);
#17409=AXIS2_PLACEMENT_3D('',#24556,#19349,#19350);
#17410=AXIS2_PLACEMENT_3D('',#24557,#19351,#19352);
#17411=AXIS2_PLACEMENT_3D('',#24558,#19353,#19354);
#17412=AXIS2_PLACEMENT_3D('',#24559,#19355,#19356);
#17413=AXIS2_PLACEMENT_3D('',#24560,#19357,#19358);
#17414=AXIS2_PLACEMENT_3D('',#24561,#19359,#19360);
#17415=AXIS2_PLACEMENT_3D('',#24562,#19361,#19362);
#17416=AXIS2_PLACEMENT_3D('',#24563,#19363,#19364);
#17417=AXIS2_PLACEMENT_3D('',#24564,#19365,#19366);
#17418=AXIS2_PLACEMENT_3D('',#24565,#19367,#19368);
#17419=AXIS2_PLACEMENT_3D('',#24566,#19369,#19370);
#17420=AXIS2_PLACEMENT_3D('',#24567,#19371,#19372);
#17421=AXIS2_PLACEMENT_3D('',#24568,#19373,#19374);
#17422=AXIS2_PLACEMENT_3D('',#24569,#19375,#19376);
#17423=AXIS2_PLACEMENT_3D('',#24570,#19377,#19378);
#17424=AXIS2_PLACEMENT_3D('',#24571,#19379,#19380);
#17425=AXIS2_PLACEMENT_3D('',#24572,#19381,#19382);
#17426=AXIS2_PLACEMENT_3D('',#24573,#19383,#19384);
#17427=AXIS2_PLACEMENT_3D('',#24574,#19385,#19386);
#17428=AXIS2_PLACEMENT_3D('',#24575,#19387,#19388);
#17429=AXIS2_PLACEMENT_3D('',#24576,#19389,#19390);
#17430=AXIS2_PLACEMENT_3D('',#24577,#19391,#19392);
#17431=AXIS2_PLACEMENT_3D('',#24578,#19393,#19394);
#17432=AXIS2_PLACEMENT_3D('',#24579,#19395,#19396);
#17433=AXIS2_PLACEMENT_3D('',#24580,#19397,#19398);
#17434=AXIS2_PLACEMENT_3D('',#24581,#19399,#19400);
#17435=AXIS2_PLACEMENT_3D('',#24582,#19401,#19402);
#17436=AXIS2_PLACEMENT_3D('',#24583,#19403,#19404);
#17437=AXIS2_PLACEMENT_3D('',#24584,#19405,#19406);
#17438=AXIS2_PLACEMENT_3D('',#24585,#19407,#19408);
#17439=AXIS2_PLACEMENT_3D('',#24586,#19409,#19410);
#17440=AXIS2_PLACEMENT_3D('',#24587,#19411,#19412);
#17441=AXIS2_PLACEMENT_3D('',#24588,#19413,#19414);
#17442=AXIS2_PLACEMENT_3D('',#24589,#19415,#19416);
#17443=AXIS2_PLACEMENT_3D('',#24590,#19417,#19418);
#17444=AXIS2_PLACEMENT_3D('',#24591,#19419,#19420);
#17445=AXIS2_PLACEMENT_3D('',#24592,#19421,#19422);
#17446=AXIS2_PLACEMENT_3D('',#24593,#19423,#19424);
#17447=AXIS2_PLACEMENT_3D('',#24594,#19425,#19426);
#17448=AXIS2_PLACEMENT_3D('',#24595,#19427,#19428);
#17449=AXIS2_PLACEMENT_3D('',#24596,#19429,#19430);
#17450=AXIS2_PLACEMENT_3D('',#24598,#19432,#19433);
#17451=AXIS2_PLACEMENT_3D('',#24600,#19435,#19436);
#17452=AXIS2_PLACEMENT_3D('',#24602,#19438,#19439);
#17453=AXIS2_PLACEMENT_3D('',#24604,#19441,#19442);
#17454=AXIS2_PLACEMENT_3D('',#24606,#19444,#19445);
#17455=AXIS2_PLACEMENT_3D('',#24608,#19447,#19448);
#17456=AXIS2_PLACEMENT_3D('',#24611,#19450,#19451);
#17457=AXIS2_PLACEMENT_3D('',#24612,#19452,#19453);
#17458=AXIS2_PLACEMENT_3D('',#24614,#19454,#19455);
#17459=AXIS2_PLACEMENT_3D('',#24615,#19456,#19457);
#17460=AXIS2_PLACEMENT_3D('',#24618,#19459,#19460);
#17461=AXIS2_PLACEMENT_3D('',#24619,#19461,#19462);
#17462=AXIS2_PLACEMENT_3D('',#24620,#19463,#19464);
#17463=AXIS2_PLACEMENT_3D('',#24622,#19465,#19466);
#17464=AXIS2_PLACEMENT_3D('',#24623,#19467,#19468);
#17465=AXIS2_PLACEMENT_3D('',#24625,#19470,#19471);
#17466=AXIS2_PLACEMENT_3D('',#24627,#19473,#19474);
#17467=AXIS2_PLACEMENT_3D('',#24628,#19475,#19476);
#17468=AXIS2_PLACEMENT_3D('',#24629,#19477,#19478);
#17469=AXIS2_PLACEMENT_3D('',#24631,#19480,#19481);
#17470=AXIS2_PLACEMENT_3D('',#24633,#19483,#19484);
#17471=AXIS2_PLACEMENT_3D('',#24635,#19486,#19487);
#17472=AXIS2_PLACEMENT_3D('',#24638,#19490,#19491);
#17473=AXIS2_PLACEMENT_3D('',#24639,#19492,#19493);
#17474=AXIS2_PLACEMENT_3D('',#24640,#19494,#19495);
#17475=AXIS2_PLACEMENT_3D('',#24641,#19496,#19497);
#17476=AXIS2_PLACEMENT_3D('',#24642,#19498,#19499);
#17477=AXIS2_PLACEMENT_3D('',#24643,#19500,#19501);
#17478=AXIS2_PLACEMENT_3D('',#24645,#19503,#19504);
#17479=AXIS2_PLACEMENT_3D('',#24646,#19505,#19506);
#17480=AXIS2_PLACEMENT_3D('',#24647,#19507,#19508);
#17481=AXIS2_PLACEMENT_3D('',#24649,#19510,#19511);
#17482=AXIS2_PLACEMENT_3D('',#24651,#19513,#19514);
#17483=AXIS2_PLACEMENT_3D('',#24653,#19516,#19517);
#17484=AXIS2_PLACEMENT_3D('',#24654,#19518,#19519);
#18791=DIRECTION('axis',(0.,0.,1.));
#18792=DIRECTION('refdir',(1.,0.,0.));
#18793=DIRECTION('center_axis',(0.331061386243095,0.943609219189173,0.));
#18794=DIRECTION('ref_axis',(0.,0.,1.));
#18795=DIRECTION('',(0.,0.,1.));
#18796=DIRECTION('',(-0.943609219189173,0.331061386243095,0.));
#18797=DIRECTION('',(0.,0.,-1.));
#18798=DIRECTION('center_axis',(0.,1.,0.));
#18799=DIRECTION('ref_axis',(-1.,0.,0.));
#18800=DIRECTION('',(-1.,0.,0.));
#18801=DIRECTION('',(-1.,0.,0.));
#18802=DIRECTION('',(0.,0.,1.));
#18803=DIRECTION('',(0.,0.,1.));
#18804=DIRECTION('',(-1.,0.,0.));
#18805=DIRECTION('',(0.,0.,-1.));
#18806=DIRECTION('center_axis',(-0.331061386243095,0.943609219189173,0.));
#18807=DIRECTION('ref_axis',(0.,0.,1.));
#18808=DIRECTION('',(0.,0.,1.));
#18809=DIRECTION('',(-0.943609219189173,-0.331061386243095,0.));
#18810=DIRECTION('center_axis',(0.,0.,1.));
#18811=DIRECTION('ref_axis',(1.,0.,0.));
#18812=DIRECTION('center_axis',(0.,0.,1.));
#18813=DIRECTION('ref_axis',(1.,0.,0.));
#18814=DIRECTION('',(0.,0.,1.));
#18815=DIRECTION('center_axis',(0.,0.,-1.));
#18816=DIRECTION('ref_axis',(0.,1.,0.));
#18817=DIRECTION('center_axis',(0.,0.,1.));
#18818=DIRECTION('ref_axis',(1.,0.,0.));
#18819=DIRECTION('center_axis',(0.,0.,-1.));
#18820=DIRECTION('ref_axis',(0.,1.,0.));
#18821=DIRECTION('center_axis',(-0.331061386243095,-0.943609219189173,0.));
#18822=DIRECTION('ref_axis',(0.,0.,-1.));
#18823=DIRECTION('',(0.,0.,1.));
#18824=DIRECTION('',(0.943609219189173,-0.331061386243095,0.));
#18825=DIRECTION('',(0.,0.,-1.));
#18826=DIRECTION('center_axis',(0.,-1.,0.));
#18827=DIRECTION('ref_axis',(1.,0.,0.));
#18828=DIRECTION('',(1.,0.,0.));
#18829=DIRECTION('',(1.,0.,0.));
#18830=DIRECTION('',(0.,0.,1.));
#18831=DIRECTION('',(0.,0.,1.));
#18832=DIRECTION('',(1.,0.,0.));
#18833=DIRECTION('',(0.,0.,-1.));
#18834=DIRECTION('center_axis',(0.331061386243095,-0.943609219189173,0.));
#18835=DIRECTION('ref_axis',(0.,0.,-1.));
#18836=DIRECTION('',(0.,0.,1.));
#18837=DIRECTION('',(0.943609219189173,0.331061386243095,0.));
#18838=DIRECTION('center_axis',(0.,0.,1.));
#18839=DIRECTION('ref_axis',(1.,0.,0.));
#18840=DIRECTION('center_axis',(0.,0.,1.));
#18841=DIRECTION('ref_axis',(1.,0.,0.));
#18842=DIRECTION('',(0.,0.,1.));
#18843=DIRECTION('center_axis',(0.,0.,-1.));
#18844=DIRECTION('ref_axis',(0.,-1.,0.));
#18845=DIRECTION('center_axis',(0.,0.,1.));
#18846=DIRECTION('ref_axis',(1.,0.,0.));
#18847=DIRECTION('center_axis',(0.,0.,-1.));
#18848=DIRECTION('ref_axis',(0.,-1.,0.));
#18849=DIRECTION('center_axis',(0.,0.,-1.));
#18850=DIRECTION('ref_axis',(1.,0.,0.));
#18851=DIRECTION('center_axis',(0.,0.,-1.));
#18852=DIRECTION('ref_axis',(1.,0.,0.));
#18853=DIRECTION('',(0.707106781186547,-8.65956056235493E-17,0.707106781186547));
#18854=DIRECTION('center_axis',(0.,0.,1.));
#18855=DIRECTION('ref_axis',(1.,0.,0.));
#18856=DIRECTION('center_axis',(0.,0.,1.));
#18857=DIRECTION('ref_axis',(0.707106781186548,0.707106781186548,0.));
#18858=DIRECTION('',(0.,1.,0.));
#18859=DIRECTION('center_axis',(0.,0.,1.));
#18860=DIRECTION('ref_axis',(0.707106781186548,-0.707106781186547,0.));
#18861=DIRECTION('',(1.,0.,0.));
#18862=DIRECTION('center_axis',(0.,0.,1.));
#18863=DIRECTION('ref_axis',(-0.707106781186548,-0.707106781186548,0.));
#18864=DIRECTION('',(0.,-1.,0.));
#18865=DIRECTION('center_axis',(0.,0.,1.));
#18866=DIRECTION('ref_axis',(-0.707106781186548,0.707106781186548,0.));
#18867=DIRECTION('',(-1.,0.,0.));
#18868=DIRECTION('center_axis',(0.,0.,-1.));
#18869=DIRECTION('ref_axis',(1.,0.,0.));
#18870=DIRECTION('center_axis',(0.,0.,1.));
#18871=DIRECTION('ref_axis',(1.,0.,0.));
#18872=DIRECTION('center_axis',(0.,0.,-1.));
#18873=DIRECTION('ref_axis',(1.,0.,0.));
#18874=DIRECTION('',(0.707106781186547,-8.65956056235493E-17,0.707106781186547));
#18875=DIRECTION('center_axis',(0.,0.,1.));
#18876=DIRECTION('ref_axis',(1.,0.,0.));
#18877=DIRECTION('center_axis',(0.,0.,1.));
#18878=DIRECTION('ref_axis',(1.,0.,0.));
#18879=DIRECTION('',(0.707106781186541,8.65956056235486E-17,-0.707106781186554));
#18880=DIRECTION('center_axis',(0.,0.,-1.));
#18881=DIRECTION('ref_axis',(1.,0.,0.));
#18882=DIRECTION('center_axis',(0.,0.,1.));
#18883=DIRECTION('ref_axis',(1.,0.,0.));
#18884=DIRECTION('',(0.,-1.,0.));
#18885=DIRECTION('center_axis',(0.,0.,-1.));
#18886=DIRECTION('ref_axis',(0.707106781186548,0.707106781186548,0.));
#18887=DIRECTION('',(1.,0.,0.));
#18888=DIRECTION('center_axis',(0.,0.,-1.));
#18889=DIRECTION('ref_axis',(-0.707106781186548,0.707106781186548,0.));
#18890=DIRECTION('',(0.,1.,0.));
#18891=DIRECTION('center_axis',(0.,0.,-1.));
#18892=DIRECTION('ref_axis',(-0.707106781186548,-0.707106781186548,0.));
#18893=DIRECTION('',(-1.,0.,0.));
#18894=DIRECTION('center_axis',(0.,0.,-1.));
#18895=DIRECTION('ref_axis',(0.707106781186548,-0.707106781186547,0.));
#18896=DIRECTION('center_axis',(0.,0.,1.));
#18897=DIRECTION('ref_axis',(1.,0.,0.));
#18898=DIRECTION('center_axis',(0.,0.,-1.));
#18899=DIRECTION('ref_axis',(1.,0.,0.));
#18900=DIRECTION('center_axis',(0.,0.,-1.));
#18901=DIRECTION('ref_axis',(1.,0.,0.));
#18902=DIRECTION('',(0.,0.,-1.));
#18903=DIRECTION('center_axis',(0.,0.,-1.));
#18904=DIRECTION('ref_axis',(1.,0.,0.));
#18905=DIRECTION('center_axis',(0.,0.,1.));
#18906=DIRECTION('ref_axis',(1.,0.,0.));
#18907=DIRECTION('',(0.707106781186541,8.65956056235486E-17,-0.707106781186554));
#18908=DIRECTION('center_axis',(0.,0.,-1.));
#18909=DIRECTION('ref_axis',(1.,0.,0.));
#18910=DIRECTION('center_axis',(0.,0.,-1.));
#18911=DIRECTION('ref_axis',(1.,0.,0.));
#18912=DIRECTION('',(0.,0.,-1.));
#18913=DIRECTION('center_axis',(0.,0.,-1.));
#18914=DIRECTION('ref_axis',(1.,0.,0.));
#18915=DIRECTION('center_axis',(1.,0.,0.));
#18916=DIRECTION('ref_axis',(0.,0.,-1.));
#18917=DIRECTION('center_axis',(1.,0.,0.));
#18918=DIRECTION('ref_axis',(0.,1.,1.41638472441199E-16));
#18919=DIRECTION('center_axis',(-1.,0.,0.));
#18920=DIRECTION('ref_axis',(0.,1.,1.41638472441199E-16));
#18921=DIRECTION('center_axis',(-1.,0.,0.));
#18922=DIRECTION('ref_axis',(0.,1.,0.));
#18923=DIRECTION('center_axis',(1.,0.,0.));
#18924=DIRECTION('ref_axis',(0.,0.,-1.));
#18925=DIRECTION('center_axis',(1.,0.,0.));
#18926=DIRECTION('ref_axis',(0.,0.,-1.));
#18927=DIRECTION('center_axis',(1.,0.,0.));
#18928=DIRECTION('ref_axis',(0.,-1.,3.06161699786838E-17));
#18929=DIRECTION('center_axis',(-1.,0.,0.));
#18930=DIRECTION('ref_axis',(0.,-1.,3.06161699786838E-17));
#18931=DIRECTION('center_axis',(-1.,0.,0.));
#18932=DIRECTION('ref_axis',(0.,-1.,3.06161699786838E-17));
#18933=DIRECTION('center_axis',(-1.,0.,0.));
#18934=DIRECTION('ref_axis',(0.,-1.,1.22464679914735E-16));
#18935=DIRECTION('center_axis',(1.,0.,0.));
#18936=DIRECTION('ref_axis',(0.,0.,-1.));
#18937=DIRECTION('center_axis',(1.,0.,0.));
#18938=DIRECTION('ref_axis',(0.,0.,-1.));
#18939=DIRECTION('center_axis',(-1.,0.,0.));
#18940=DIRECTION('ref_axis',(0.,-1.,1.83697019872103E-16));
#18941=DIRECTION('center_axis',(0.,-1.,-1.22464679914735E-16));
#18942=DIRECTION('ref_axis',(0.,-1.22464679914735E-16,1.));
#18943=DIRECTION('center_axis',(1.,0.,0.));
#18944=DIRECTION('ref_axis',(0.,-1.,3.06161699786838E-17));
#18945=DIRECTION('center_axis',(1.,0.,0.));
#18946=DIRECTION('ref_axis',(0.,-1.,3.06161699786838E-17));
#18947=DIRECTION('center_axis',(-1.,0.,0.));
#18948=DIRECTION('ref_axis',(0.,1.,0.));
#18949=DIRECTION('',(-0.64018439966448,-0.768221279597376,-9.4079973109581E-17));
#18950=DIRECTION('center_axis',(1.,0.,0.));
#18951=DIRECTION('ref_axis',(0.,1.,0.));
#18952=DIRECTION('center_axis',(1.,0.,0.));
#18953=DIRECTION('ref_axis',(0.,1.,0.));
#18954=DIRECTION('center_axis',(1.,0.,0.));
#18955=DIRECTION('ref_axis',(0.,0.,-1.));
#18956=DIRECTION('',(0.,-1.77635683940025E-16,-1.));
#18957=DIRECTION('',(0.,-1.,0.));
#18958=DIRECTION('',(0.,1.99840144432528E-16,1.));
#18959=DIRECTION('',(0.,1.,0.));
#18960=DIRECTION('',(0.,0.866025403784439,0.5));
#18961=DIRECTION('',(0.,0.5,-0.866025403784438));
#18962=DIRECTION('',(0.,-0.866025403784439,-0.5));
#18963=DIRECTION('',(0.,-0.5,0.866025403784439));
#18964=DIRECTION('',(0.,6.66133814775094E-17,1.));
#18965=DIRECTION('',(0.,1.,0.));
#18966=DIRECTION('',(0.,-7.7715611723761E-17,-1.));
#18967=DIRECTION('',(0.,-1.,0.));
#18968=DIRECTION('',(0.,-0.866025403784439,0.5));
#18969=DIRECTION('',(0.,0.5,0.866025403784438));
#18970=DIRECTION('',(0.,0.866025403784439,-0.5));
#18971=DIRECTION('',(0.,-0.5,-0.866025403784439));
#18972=DIRECTION('',(0.,-0.866025403784439,-0.5));
#18973=DIRECTION('',(0.,-0.499999999999999,0.866025403784439));
#18974=DIRECTION('',(0.,0.866025403784439,0.5));
#18975=DIRECTION('',(0.,0.5,-0.866025403784439));
#18976=DIRECTION('',(0.,0.866025403784438,-0.5));
#18977=DIRECTION('',(0.,-0.500000000000001,-0.866025403784438));
#18978=DIRECTION('',(0.,-0.866025403784438,0.5));
#18979=DIRECTION('',(0.,0.5,0.866025403784438));
#18980=DIRECTION('center_axis',(1.,0.,0.));
#18981=DIRECTION('ref_axis',(0.,-0.999985032132206,0.00547133544502502));
#18982=DIRECTION('center_axis',(-1.,0.,0.));
#18983=DIRECTION('ref_axis',(0.,-0.999998948230417,0.00145035790781154));
#18984=DIRECTION('center_axis',(-1.,0.,0.));
#18985=DIRECTION('ref_axis',(0.,0.999955202286269,-0.00946538011005637));
#18986=DIRECTION('center_axis',(1.,0.,0.));
#18987=DIRECTION('ref_axis',(0.,0.,-1.));
#18988=DIRECTION('',(0.,1.,0.));
#18989=DIRECTION('',(0.,0.,1.));
#18990=DIRECTION('',(0.,0.,1.));
#18991=DIRECTION('',(0.,-1.,0.));
#18992=DIRECTION('center_axis',(-1.,0.,0.));
#18993=DIRECTION('ref_axis',(0.,0.,-1.));
#18994=DIRECTION('center_axis',(-1.,0.,0.));
#18995=DIRECTION('ref_axis',(0.,0.,-1.));
#18996=DIRECTION('center_axis',(-1.,0.,0.));
#18997=DIRECTION('ref_axis',(0.,0.,-1.));
#18998=DIRECTION('center_axis',(1.,0.,0.));
#18999=DIRECTION('ref_axis',(0.,0.,-1.));
#19000=DIRECTION('center_axis',(1.,0.,0.));
#19001=DIRECTION('ref_axis',(0.,-0.999998948230417,0.00145035790781157));
#19002=DIRECTION('center_axis',(1.,0.,0.));
#19003=DIRECTION('ref_axis',(0.,-0.999998948230417,0.00145035790781157));
#19004=DIRECTION('center_axis',(1.,0.,0.));
#19005=DIRECTION('ref_axis',(0.,1.,0.));
#19006=DIRECTION('center_axis',(-1.,0.,0.));
#19007=DIRECTION('ref_axis',(0.,1.,0.));
#19008=DIRECTION('center_axis',(1.,0.,0.));
#19009=DIRECTION('ref_axis',(0.,0.999998948230416,0.00145035790796071));
#19010=DIRECTION('center_axis',(-1.,0.,0.));
#19011=DIRECTION('ref_axis',(0.,1.,0.));
#19012=DIRECTION('',(-1.,0.,0.));
#19013=DIRECTION('center_axis',(-1.,0.,0.));
#19014=DIRECTION('ref_axis',(0.,1.,1.22464679914735E-16));
#19015=DIRECTION('center_axis',(1.,0.,0.));
#19016=DIRECTION('ref_axis',(0.,0.999985032132206,0.00547133544502336));
#19017=DIRECTION('center_axis',(-1.,0.,0.));
#19018=DIRECTION('ref_axis',(0.,0.999998948230416,0.00145035790796071));
#19019=DIRECTION('center_axis',(-1.,0.,0.));
#19020=DIRECTION('ref_axis',(0.,-0.999955202286269,-0.00946538011005535));
#19021=DIRECTION('center_axis',(1.,0.,0.));
#19022=DIRECTION('ref_axis',(0.,0.,-1.));
#19023=DIRECTION('',(0.,-1.,0.));
#19024=DIRECTION('',(0.,0.,-1.));
#19025=DIRECTION('',(0.,0.,-1.));
#19026=DIRECTION('',(0.,1.,0.));
#19027=DIRECTION('center_axis',(-1.,0.,0.));
#19028=DIRECTION('ref_axis',(0.,0.,-1.));
#19029=DIRECTION('center_axis',(-1.,0.,0.));
#19030=DIRECTION('ref_axis',(0.,0.,-1.));
#19031=DIRECTION('center_axis',(-1.,0.,0.));
#19032=DIRECTION('ref_axis',(0.,0.,-1.));
#19033=DIRECTION('center_axis',(-1.,0.,0.));
#19034=DIRECTION('ref_axis',(0.,0.,1.));
#19035=DIRECTION('center_axis',(1.,0.,0.));
#19036=DIRECTION('ref_axis',(0.,1.,1.22464679914735E-16));
#19037=DIRECTION('center_axis',(0.,0.,-1.));
#19038=DIRECTION('ref_axis',(0.,-1.,0.));
#19039=DIRECTION('center_axis',(1.,0.,0.));
#19040=DIRECTION('ref_axis',(0.,1.,1.22464679914735E-16));
#19041=DIRECTION('center_axis',(-1.,0.,0.));
#19042=DIRECTION('ref_axis',(0.,0.,1.));
#19043=DIRECTION('center_axis',(1.,0.,0.));
#19044=DIRECTION('ref_axis',(0.,0.,-1.));
#19045=DIRECTION('center_axis',(1.,0.,0.));
#19046=DIRECTION('ref_axis',(0.,0.,-1.));
#19047=DIRECTION('center_axis',(1.,0.,0.));
#19048=DIRECTION('ref_axis',(0.,0.,-1.));
#19049=DIRECTION('center_axis',(1.,0.,0.));
#19050=DIRECTION('ref_axis',(0.,0.,-1.));
#19051=DIRECTION('center_axis',(1.,0.,0.));
#19052=DIRECTION('ref_axis',(0.,0.,-1.));
#19053=DIRECTION('center_axis',(1.,0.,0.));
#19054=DIRECTION('ref_axis',(0.,0.,-1.));
#19055=DIRECTION('center_axis',(-1.,0.,0.));
#19056=DIRECTION('ref_axis',(0.,1.,0.));
#19057=DIRECTION('center_axis',(0.,0.,1.));
#19058=DIRECTION('ref_axis',(1.,0.,0.));
#19059=DIRECTION('center_axis',(0.,0.,1.));
#19060=DIRECTION('ref_axis',(-0.309915766398542,-0.950764017902237,0.));
#19061=DIRECTION('center_axis',(-1.,0.,0.));
#19062=DIRECTION('ref_axis',(0.,0.,-1.));
#19063=DIRECTION('center_axis',(0.,0.,-1.));
#19064=DIRECTION('ref_axis',(-0.309915766398542,-0.950764017902237,0.));
#19065=DIRECTION('center_axis',(1.,0.,0.));
#19066=DIRECTION('ref_axis',(0.,-0.707106781186546,-0.707106781186549));
#19067=DIRECTION('center_axis',(-1.,0.,0.));
#19068=DIRECTION('ref_axis',(0.,0.,-1.));
#19069=DIRECTION('',(-1.,0.,0.));
#19070=DIRECTION('',(1.,0.,0.));
#19071=DIRECTION('center_axis',(0.,0.,1.));
#19072=DIRECTION('ref_axis',(1.,0.,0.));
#19073=DIRECTION('center_axis',(0.,-1.,0.));
#19074=DIRECTION('ref_axis',(0.,0.,-1.));
#19075=DIRECTION('center_axis',(0.,0.,-1.));
#19076=DIRECTION('ref_axis',(0.707106781186548,-0.707106781186547,0.));
#19077=DIRECTION('center_axis',(0.,0.,1.));
#19078=DIRECTION('ref_axis',(0.707106781186548,-0.707106781186547,0.));
#19079=DIRECTION('center_axis',(0.,1.,0.));
#19080=DIRECTION('ref_axis',(0.707106781186544,0.,-0.707106781186551));
#19081=DIRECTION('',(0.,-1.,0.));
#19082=DIRECTION('',(0.,1.,0.));
#19083=DIRECTION('center_axis',(1.,0.,0.));
#19084=DIRECTION('ref_axis',(0.,1.,0.));
#19085=DIRECTION('',(0.,0.,1.));
#19086=DIRECTION('',(0.,0.,1.));
#19087=DIRECTION('',(0.,-1.,0.));
#19088=DIRECTION('',(0.,0.,1.));
#19089=DIRECTION('',(0.,1.,0.));
#19090=DIRECTION('',(0.,0.,1.));
#19091=DIRECTION('center_axis',(0.,0.,1.));
#19092=DIRECTION('ref_axis',(1.,0.,0.));
#19093=DIRECTION('center_axis',(0.,0.,-1.));
#19094=DIRECTION('ref_axis',(-1.,0.,0.));
#19095=DIRECTION('',(-1.,0.,0.));
#19096=DIRECTION('center_axis',(0.,0.,-1.));
#19097=DIRECTION('ref_axis',(2.22044604925031E-15,-1.,0.));
#19098=DIRECTION('center_axis',(0.,1.,0.));
#19099=DIRECTION('ref_axis',(0.707106781186544,0.,0.707106781186551));
#19100=DIRECTION('center_axis',(0.,1.,0.));
#19101=DIRECTION('ref_axis',(0.,0.,1.));
#19102=DIRECTION('center_axis',(0.,-1.,0.));
#19103=DIRECTION('ref_axis',(1.,0.,0.));
#19104=DIRECTION('center_axis',(0.,0.,1.));
#19105=DIRECTION('ref_axis',(1.,0.,0.));
#19106=DIRECTION('center_axis',(1.,0.,0.));
#19107=DIRECTION('ref_axis',(0.,1.,0.));
#19108=DIRECTION('center_axis',(0.,0.,1.));
#19109=DIRECTION('ref_axis',(0.707106781186548,0.707106781186548,0.));
#19110=DIRECTION('center_axis',(-1.,0.,0.));
#19111=DIRECTION('ref_axis',(0.,0.707106781186549,0.707106781186546));
#19112=DIRECTION('center_axis',(1.,0.,0.));
#19113=DIRECTION('ref_axis',(0.,1.,0.));
#19114=DIRECTION('',(-1.,0.,0.));
#19115=DIRECTION('center_axis',(0.,0.,1.));
#19116=DIRECTION('ref_axis',(1.,0.,0.));
#19117=DIRECTION('center_axis',(0.,1.,0.));
#19118=DIRECTION('ref_axis',(-1.,0.,0.));
#19119=DIRECTION('center_axis',(0.,0.,1.));
#19120=DIRECTION('ref_axis',(-0.707106781186548,0.707106781186548,0.));
#19121=DIRECTION('center_axis',(0.,-1.,0.));
#19122=DIRECTION('ref_axis',(-0.707106781186548,0.,0.707106781186548));
#19123=DIRECTION('center_axis',(0.,1.,0.));
#19124=DIRECTION('ref_axis',(-1.,0.,0.));
#19125=DIRECTION('',(0.,-1.,0.));
#19126=DIRECTION('center_axis',(0.,0.,1.));
#19127=DIRECTION('ref_axis',(1.,0.,0.));
#19128=DIRECTION('center_axis',(-1.,0.,0.));
#19129=DIRECTION('ref_axis',(0.,-1.,0.));
#19130=DIRECTION('center_axis',(0.,0.,1.));
#19131=DIRECTION('ref_axis',(-0.707106781186548,-0.707106781186548,0.));
#19132=DIRECTION('center_axis',(1.,0.,0.));
#19133=DIRECTION('ref_axis',(0.,-0.707106781186549,0.707106781186546));
#19134=DIRECTION('center_axis',(-1.,0.,0.));
#19135=DIRECTION('ref_axis',(0.,-1.,0.));
#19136=DIRECTION('',(1.,0.,0.));
#19137=DIRECTION('center_axis',(0.,0.,1.));
#19138=DIRECTION('ref_axis',(1.,0.,0.));
#19139=DIRECTION('center_axis',(0.,0.,1.));
#19140=DIRECTION('ref_axis',(0.707106781186548,-0.707106781186547,0.));
#19141=DIRECTION('center_axis',(0.,0.,1.));
#19142=DIRECTION('ref_axis',(0.,1.,0.));
#19143=DIRECTION('',(0.,0.,1.));
#19144=DIRECTION('center_axis',(0.,0.,-1.));
#19145=DIRECTION('ref_axis',(-0.309915766398542,0.950764017902237,0.));
#19146=DIRECTION('',(0.,0.,1.));
#19147=DIRECTION('center_axis',(0.,1.,0.));
#19148=DIRECTION('ref_axis',(-1.,0.,0.));
#19149=DIRECTION('',(0.,0.,1.));
#19150=DIRECTION('',(1.,0.,0.));
#19151=DIRECTION('center_axis',(0.,0.,1.));
#19152=DIRECTION('ref_axis',(1.,5.55111512312578E-16,0.));
#19153=DIRECTION('center_axis',(0.,0.,-1.));
#19154=DIRECTION('ref_axis',(0.707106781186548,0.707106781186548,0.));
#19155=DIRECTION('center_axis',(0.,1.,0.));
#19156=DIRECTION('ref_axis',(0.707106781186544,0.,-0.707106781186551));
#19157=DIRECTION('center_axis',(0.,-1.,0.));
#19158=DIRECTION('ref_axis',(0.,0.,-1.));
#19159=DIRECTION('',(0.,1.,0.));
#19160=DIRECTION('center_axis',(-1.,0.,0.));
#19161=DIRECTION('ref_axis',(0.,0.707106781186546,-0.707106781186549));
#19162=DIRECTION('center_axis',(-1.,0.,0.));
#19163=DIRECTION('ref_axis',(0.,1.,0.));
#19164=DIRECTION('',(-1.,0.,0.));
#19165=DIRECTION('center_axis',(1.,0.,0.));
#19166=DIRECTION('ref_axis',(0.,0.,-1.));
#19167=DIRECTION('center_axis',(0.,0.,1.));
#19168=DIRECTION('ref_axis',(1.,0.,0.));
#19169=DIRECTION('center_axis',(0.,0.,1.));
#19170=DIRECTION('ref_axis',(-0.309915766398542,0.950764017902237,0.));
#19171=DIRECTION('center_axis',(0.,0.,1.));
#19172=DIRECTION('ref_axis',(1.,0.,0.));
#19173=DIRECTION('center_axis',(0.,0.,1.));
#19174=DIRECTION('ref_axis',(0.707106781186548,0.707106781186548,0.));
#19175=DIRECTION('center_axis',(0.,0.,1.));
#19176=DIRECTION('ref_axis',(1.,0.,0.));
#19177=DIRECTION('center_axis',(0.,0.,-1.));
#19178=DIRECTION('ref_axis',(1.,5.55111512312577E-16,0.));
#19179=DIRECTION('',(1.,0.,0.));
#19180=DIRECTION('center_axis',(0.,0.,-1.));
#19181=DIRECTION('ref_axis',(0.,1.,0.));
#19182=DIRECTION('center_axis',(1.,0.,0.));
#19183=DIRECTION('ref_axis',(0.,0.,-1.));
#19184=DIRECTION('center_axis',(0.,-1.,-1.22464679914735E-16));
#19185=DIRECTION('ref_axis',(0.,-1.22464679914735E-16,1.));
#19186=DIRECTION('center_axis',(1.,0.,0.));
#19187=DIRECTION('ref_axis',(0.,1.,6.12323399573677E-17));
#19188=DIRECTION('center_axis',(1.,0.,0.));
#19189=DIRECTION('ref_axis',(0.,1.,6.12323399573677E-17));
#19190=DIRECTION('center_axis',(-1.,0.,0.));
#19191=DIRECTION('ref_axis',(0.,1.,0.));
#19192=DIRECTION('',(0.888217643155949,0.459422918873766,5.62630807053692E-17));
#19193=DIRECTION('center_axis',(1.,0.,0.));
#19194=DIRECTION('ref_axis',(0.,0.,-1.));
#19195=DIRECTION('center_axis',(0.,0.,-1.));
#19196=DIRECTION('ref_axis',(-0.816496580927725,0.577350269189627,0.));
#19197=DIRECTION('',(0.,0.,-1.));
#19198=DIRECTION('',(0.,0.,1.));
#19199=DIRECTION('center_axis',(0.,0.,1.));
#19200=DIRECTION('ref_axis',(-0.816496580927725,-0.577350269189627,0.));
#19201=DIRECTION('',(0.,0.,-1.));
#19202=DIRECTION('',(0.,0.,1.));
#19203=DIRECTION('center_axis',(1.,0.,0.));
#19204=DIRECTION('ref_axis',(0.,0.,-1.));
#19205=DIRECTION('center_axis',(1.,0.,0.));
#19206=DIRECTION('ref_axis',(0.,0.,-1.));
#19207=DIRECTION('center_axis',(1.,0.,0.));
#19208=DIRECTION('ref_axis',(0.,0.,-1.));
#19209=DIRECTION('center_axis',(0.,0.,1.));
#19210=DIRECTION('ref_axis',(1.,0.,0.));
#19211=DIRECTION('center_axis',(0.,0.,1.));
#19212=DIRECTION('ref_axis',(1.,0.,0.));
#19213=DIRECTION('',(0.,0.,1.));
#19214=DIRECTION('',(0.,0.,1.));
#19215=DIRECTION('center_axis',(0.,0.,1.));
#19216=DIRECTION('ref_axis',(1.,0.,0.));
#19217=DIRECTION('center_axis',(0.,0.,1.));
#19218=DIRECTION('ref_axis',(1.,0.,0.));
#19219=DIRECTION('center_axis',(0.,0.,1.));
#19220=DIRECTION('ref_axis',(-0.294281086116927,-0.955718913883074,0.));
#19221=DIRECTION('center_axis',(-1.,0.,0.));
#19222=DIRECTION('ref_axis',(0.,-1.,0.));
#19223=DIRECTION('center_axis',(0.,0.,-1.));
#19224=DIRECTION('ref_axis',(-0.294281086116927,-0.955718913883074,0.));
#19225=DIRECTION('center_axis',(1.,0.,0.));
#19226=DIRECTION('ref_axis',(0.,-0.707106781186549,0.707106781186546));
#19227=DIRECTION('',(-1.,0.,0.));
#19228=DIRECTION('',(1.,0.,0.));
#19229=DIRECTION('center_axis',(-1.,0.,0.));
#19230=DIRECTION('ref_axis',(0.,-1.,0.));
#19231=DIRECTION('',(-1.,0.,0.));
#19232=DIRECTION('center_axis',(0.,0.,1.));
#19233=DIRECTION('ref_axis',(1.,0.,0.));
#19234=DIRECTION('center_axis',(0.,-1.,0.));
#19235=DIRECTION('ref_axis',(1.,0.,0.));
#19236=DIRECTION('center_axis',(0.,0.,-1.));
#19237=DIRECTION('ref_axis',(0.707106781186548,-0.707106781186547,0.));
#19238=DIRECTION('center_axis',(0.,0.,1.));
#19239=DIRECTION('ref_axis',(0.707106781186548,-0.707106781186547,0.));
#19240=DIRECTION('center_axis',(0.,1.,0.));
#19241=DIRECTION('ref_axis',(0.707106781186548,0.,0.707106781186548));
#19242=DIRECTION('',(0.,-1.,0.));
#19243=DIRECTION('',(0.,1.,0.));
#19244=DIRECTION('center_axis',(0.,-1.,0.));
#19245=DIRECTION('ref_axis',(1.,0.,0.));
#19246=DIRECTION('',(0.,0.,1.));
#19247=DIRECTION('',(-1.,0.,0.));
#19248=DIRECTION('',(0.,0.,1.));
#19249=DIRECTION('center_axis',(0.,0.,1.));
#19250=DIRECTION('ref_axis',(-1.,0.,0.));
#19251=DIRECTION('',(0.,0.,1.));
#19252=DIRECTION('center_axis',(0.,0.,-1.));
#19253=DIRECTION('ref_axis',(-0.707106781186548,-0.707106781186548,0.));
#19254=DIRECTION('center_axis',(0.,0.,1.));
#19255=DIRECTION('ref_axis',(1.,0.,0.));
#19256=DIRECTION('center_axis',(0.,0.,1.));
#19257=DIRECTION('ref_axis',(0.,-1.,0.));
#19258=DIRECTION('center_axis',(0.,0.,1.));
#19259=DIRECTION('ref_axis',(-1.,0.,0.));
#19260=DIRECTION('center_axis',(0.,0.,-1.));
#19261=DIRECTION('ref_axis',(0.,-1.,0.));
#19262=DIRECTION('center_axis',(0.,0.,1.));
#19263=DIRECTION('ref_axis',(0.,-1.,0.));
#19264=DIRECTION('center_axis',(0.,0.,1.));
#19265=DIRECTION('ref_axis',(1.,0.,0.));
#19266=DIRECTION('center_axis',(0.,1.,0.));
#19267=DIRECTION('ref_axis',(1.,0.,0.));
#19268=DIRECTION('center_axis',(1.,0.,0.));
#19269=DIRECTION('ref_axis',(0.,0.,-1.));
#19270=DIRECTION('center_axis',(0.,0.,-1.));
#19271=DIRECTION('ref_axis',(0.707106781186548,0.707106781186548,0.));
#19272=DIRECTION('center_axis',(-1.,0.,0.));
#19273=DIRECTION('ref_axis',(0.,0.707106781186549,-0.707106781186546));
#19274=DIRECTION('center_axis',(1.,0.,0.));
#19275=DIRECTION('ref_axis',(0.,0.,-1.));
#19276=DIRECTION('',(1.,0.,0.));
#19277=DIRECTION('center_axis',(0.,0.,1.));
#19278=DIRECTION('ref_axis',(1.,0.,0.));
#19279=DIRECTION('center_axis',(0.,1.,0.));
#19280=DIRECTION('ref_axis',(0.,0.,-1.));
#19281=DIRECTION('center_axis',(0.,0.,-1.));
#19282=DIRECTION('ref_axis',(-0.707106781186548,0.707106781186548,0.));
#19283=DIRECTION('center_axis',(0.,-1.,0.));
#19284=DIRECTION('ref_axis',(-0.707106781186551,0.,-0.707106781186544));
#19285=DIRECTION('center_axis',(0.,1.,0.));
#19286=DIRECTION('ref_axis',(0.,0.,-1.));
#19287=DIRECTION('',(0.,1.,0.));
#19288=DIRECTION('center_axis',(0.,0.,1.));
#19289=DIRECTION('ref_axis',(1.,0.,0.));
#19290=DIRECTION('center_axis',(-1.,0.,0.));
#19291=DIRECTION('ref_axis',(0.,0.,-1.));
#19292=DIRECTION('center_axis',(1.,0.,0.));
#19293=DIRECTION('ref_axis',(0.,-0.707106781186549,-0.707106781186546));
#19294=DIRECTION('center_axis',(-1.,0.,0.));
#19295=DIRECTION('ref_axis',(0.,0.,-1.));
#19296=DIRECTION('center_axis',(0.,0.,1.));
#19297=DIRECTION('ref_axis',(1.,0.,0.));
#19298=DIRECTION('center_axis',(0.,-1.,0.));
#19299=DIRECTION('ref_axis',(0.,0.,-1.));
#19300=DIRECTION('center_axis',(0.,0.,-1.));
#19301=DIRECTION('ref_axis',(0.707106781186548,-0.707106781186547,0.));
#19302=DIRECTION('center_axis',(0.,1.,0.));
#19303=DIRECTION('ref_axis',(0.707106781186548,0.,-0.707106781186548));
#19304=DIRECTION('',(0.,-1.,0.));
#19305=DIRECTION('center_axis',(0.,0.,1.));
#19306=DIRECTION('ref_axis',(1.11022302462516E-15,-1.,0.));
#19307=DIRECTION('',(0.,0.,1.));
#19308=DIRECTION('center_axis',(1.,0.,0.));
#19309=DIRECTION('ref_axis',(0.,1.,0.));
#19310=DIRECTION('',(0.,0.,1.));
#19311=DIRECTION('',(0.,1.,0.));
#19312=DIRECTION('',(0.,0.,1.));
#19313=DIRECTION('',(0.,0.,1.));
#19314=DIRECTION('center_axis',(0.,0.,1.));
#19315=DIRECTION('ref_axis',(1.,5.55111512312578E-16,0.));
#19316=DIRECTION('',(0.,0.,1.));
#19317=DIRECTION('center_axis',(0.,0.,1.));
#19318=DIRECTION('ref_axis',(0.707106781186548,0.707106781186548,0.));
#19319=DIRECTION('center_axis',(0.,1.,0.));
#19320=DIRECTION('ref_axis',(0.707106781186548,0.,0.707106781186548));
#19321=DIRECTION('center_axis',(0.,-1.,0.));
#19322=DIRECTION('ref_axis',(1.,0.,0.));
#19323=DIRECTION('',(0.,-1.,0.));
#19324=DIRECTION('center_axis',(0.,0.,1.));
#19325=DIRECTION('ref_axis',(1.,0.,0.));
#19326=DIRECTION('center_axis',(1.,0.,0.));
#19327=DIRECTION('ref_axis',(0.,1.,0.));
#19328=DIRECTION('center_axis',(0.,0.,-1.));
#19329=DIRECTION('ref_axis',(0.707106781186548,0.707106781186548,0.));
#19330=DIRECTION('center_axis',(-1.,0.,0.));
#19331=DIRECTION('ref_axis',(0.,0.707106781186549,0.707106781186546));
#19332=DIRECTION('',(1.,0.,0.));
#19333=DIRECTION('',(-1.,0.,0.));
#19334=DIRECTION('center_axis',(1.,0.,0.));
#19335=DIRECTION('ref_axis',(0.,1.,0.));
#19336=DIRECTION('',(1.,0.,0.));
#19337=DIRECTION('center_axis',(0.,0.,1.));
#19338=DIRECTION('ref_axis',(1.,0.,0.));
#19339=DIRECTION('center_axis',(0.,0.,-1.));
#19340=DIRECTION('ref_axis',(-0.294281086116927,0.955718913883074,0.));
#19341=DIRECTION('center_axis',(0.,0.,1.));
#19342=DIRECTION('ref_axis',(-0.294281086116927,0.955718913883074,0.));
#19343=DIRECTION('center_axis',(0.,0.,1.));
#19344=DIRECTION('ref_axis',(1.,0.,0.));
#19345=DIRECTION('center_axis',(0.,0.,1.));
#19346=DIRECTION('ref_axis',(0.,1.,0.));
#19347=DIRECTION('center_axis',(0.,0.,1.));
#19348=DIRECTION('ref_axis',(0.,1.,0.));
#19349=DIRECTION('center_axis',(0.,0.,1.));
#19350=DIRECTION('ref_axis',(1.,0.,0.));
#19351=DIRECTION('center_axis',(0.,0.,1.));
#19352=DIRECTION('ref_axis',(0.,1.,0.));
#19353=DIRECTION('center_axis',(0.,0.,1.));
#19354=DIRECTION('ref_axis',(1.,5.55111512312577E-16,0.));
#19355=DIRECTION('center_axis',(0.,0.,-1.));
#19356=DIRECTION('ref_axis',(0.,1.,0.));
#19357=DIRECTION('center_axis',(0.,0.,1.));
#19358=DIRECTION('ref_axis',(0.,-1.,0.));
#19359=DIRECTION('center_axis',(0.,0.,-1.));
#19360=DIRECTION('ref_axis',(0.707106781186546,-0.707106781186549,0.));
#19361=DIRECTION('center_axis',(0.,1.77635683940025E-16,1.));
#19362=DIRECTION('ref_axis',(0.707106781186546,0.707106781186549,0.));
#19363=DIRECTION('center_axis',(0.,0.,1.));
#19364=DIRECTION('ref_axis',(0.707106781186546,0.707106781186549,0.));
#19365=DIRECTION('center_axis',(0.,-0.866025403784439,-0.5));
#19366=DIRECTION('ref_axis',(0.,0.5,-0.866025403784439));
#19367=DIRECTION('center_axis',(0.,0.866025403784439,0.5));
#19368=DIRECTION('ref_axis',(0.707106781186546,0.353553390593275,-0.612372435695796));
#19369=DIRECTION('center_axis',(0.,-0.866025403784439,-0.5));
#19370=DIRECTION('ref_axis',(0.707106781186547,-0.353553390593273,0.612372435695796));
#19371=DIRECTION('center_axis',(0.,-0.866025403784439,-0.5));
#19372=DIRECTION('ref_axis',(0.707106781186547,-0.353553390593273,0.612372435695796));
#19373=DIRECTION('center_axis',(0.,0.,-1.));
#19374=DIRECTION('ref_axis',(0.,1.,0.));
#19375=DIRECTION('center_axis',(0.,0.,1.));
#19376=DIRECTION('ref_axis',(0.707106781186546,0.707106781186549,0.));
#19377=DIRECTION('center_axis',(0.,-6.66133814775094E-17,-1.));
#19378=DIRECTION('ref_axis',(0.707106781186546,-0.707106781186549,0.));
#19379=DIRECTION('center_axis',(0.,0.,-1.));
#19380=DIRECTION('ref_axis',(0.707106781186546,-0.707106781186549,0.));
#19381=DIRECTION('center_axis',(0.,0.866025403784439,-0.5));
#19382=DIRECTION('ref_axis',(0.,0.5,0.866025403784439));
#19383=DIRECTION('center_axis',(0.,-0.866025403784439,0.5));
#19384=DIRECTION('ref_axis',(0.707106781186546,0.353553390593275,0.612372435695795));
#19385=DIRECTION('center_axis',(0.,0.866025403784439,-0.5));
#19386=DIRECTION('ref_axis',(0.707106781186546,-0.353553390593273,-0.612372435695797));
#19387=DIRECTION('center_axis',(0.,0.866025403784439,-0.5));
#19388=DIRECTION('ref_axis',(0.707106781186546,-0.353553390593273,-0.612372435695797));
#19389=DIRECTION('center_axis',(0.,0.866025403784439,0.5));
#19390=DIRECTION('ref_axis',(0.,-0.5,0.866025403784439));
#19391=DIRECTION('center_axis',(0.,-0.866025403784439,-0.5));
#19392=DIRECTION('ref_axis',(0.707106781186546,-0.353553390593275,0.612372435695795));
#19393=DIRECTION('center_axis',(0.,0.866025403784439,0.5));
#19394=DIRECTION('ref_axis',(0.707106781186547,0.353553390593273,-0.612372435695796));
#19395=DIRECTION('center_axis',(0.,0.866025403784439,0.499999999999999));
#19396=DIRECTION('ref_axis',(0.707106781186547,0.353553390593273,-0.612372435695796));
#19397=DIRECTION('center_axis',(0.,-0.866025403784438,0.5));
#19398=DIRECTION('ref_axis',(0.,-0.5,-0.866025403784438));
#19399=DIRECTION('center_axis',(0.,0.866025403784438,-0.5));
#19400=DIRECTION('ref_axis',(0.707106781186546,-0.353553390593275,-0.612372435695795));
#19401=DIRECTION('center_axis',(0.,-0.866025403784438,0.5));
#19402=DIRECTION('ref_axis',(0.707106781186546,0.353553390593276,0.612372435695795));
#19403=DIRECTION('center_axis',(0.,-0.866025403784438,0.500000000000001));
#19404=DIRECTION('ref_axis',(0.707106781186546,0.353553390593276,0.612372435695795));
#19405=DIRECTION('center_axis',(0.,0.866025403784438,-0.500000000000001));
#19406=DIRECTION('ref_axis',(0.,0.500000000000001,0.866025403784438));
#19407=DIRECTION('center_axis',(0.,-0.866025403784439,-0.499999999999999));
#19408=DIRECTION('ref_axis',(0.,0.499999999999999,-0.866025403784439));
#19409=DIRECTION('center_axis',(0.,-0.866025403784439,0.5));
#19410=DIRECTION('ref_axis',(0.,-0.5,-0.866025403784438));
#19411=DIRECTION('center_axis',(0.,0.,1.));
#19412=DIRECTION('ref_axis',(0.,-1.,0.));
#19413=DIRECTION('center_axis',(0.,0.866025403784439,0.5));
#19414=DIRECTION('ref_axis',(0.,-0.5,0.866025403784438));
#19415=DIRECTION('center_axis',(0.,0.,-1.));
#19416=DIRECTION('ref_axis',(0.,1.,0.));
#19417=DIRECTION('center_axis',(0.,0.,1.));
#19418=DIRECTION('ref_axis',(1.,0.,0.));
#19419=DIRECTION('center_axis',(0.,0.,1.));
#19420=DIRECTION('ref_axis',(1.,0.,0.));
#19421=DIRECTION('center_axis',(0.,0.,1.));
#19422=DIRECTION('ref_axis',(1.,0.,0.));
#19423=DIRECTION('center_axis',(0.,0.,1.));
#19424=DIRECTION('ref_axis',(1.,0.,0.));
#19425=DIRECTION('center_axis',(0.,0.,1.));
#19426=DIRECTION('ref_axis',(1.,0.,0.));
#19427=DIRECTION('center_axis',(0.,0.,1.));
#19428=DIRECTION('ref_axis',(2.22044604925031E-15,-1.,0.));
#19429=DIRECTION('center_axis',(1.,0.,0.));
#19430=DIRECTION('ref_axis',(0.,0.,-1.));
#19431=DIRECTION('',(1.,0.,0.));
#19432=DIRECTION('center_axis',(1.,0.,0.));
#19433=DIRECTION('ref_axis',(0.,0.,-1.));
#19434=DIRECTION('',(1.,0.,0.));
#19435=DIRECTION('center_axis',(1.,0.,0.));
#19436=DIRECTION('ref_axis',(0.,0.,-1.));
#19437=DIRECTION('',(1.,0.,0.));
#19438=DIRECTION('center_axis',(1.,0.,0.));
#19439=DIRECTION('ref_axis',(0.,0.,-1.));
#19440=DIRECTION('',(1.,0.,0.));
#19441=DIRECTION('center_axis',(1.,0.,0.));
#19442=DIRECTION('ref_axis',(0.,0.,-1.));
#19443=DIRECTION('',(1.,0.,0.));
#19444=DIRECTION('center_axis',(1.,0.,0.));
#19445=DIRECTION('ref_axis',(0.,0.,-1.));
#19446=DIRECTION('',(1.,0.,0.));
#19447=DIRECTION('center_axis',(0.,0.,1.));
#19448=DIRECTION('ref_axis',(1.,0.,0.));
#19449=DIRECTION('',(0.,0.,1.));
#19450=DIRECTION('center_axis',(0.,0.,1.));
#19451=DIRECTION('ref_axis',(1.,0.,0.));
#19452=DIRECTION('center_axis',(0.,0.,1.));
#19453=DIRECTION('ref_axis',(1.,0.,0.));
#19454=DIRECTION('center_axis',(0.,0.,1.));
#19455=DIRECTION('ref_axis',(1.,0.,0.));
#19456=DIRECTION('center_axis',(0.,0.,1.));
#19457=DIRECTION('ref_axis',(1.,0.,0.));
#19458=DIRECTION('',(0.,0.,1.));
#19459=DIRECTION('center_axis',(0.,0.,1.));
#19460=DIRECTION('ref_axis',(1.,0.,0.));
#19461=DIRECTION('center_axis',(0.,0.,1.));
#19462=DIRECTION('ref_axis',(1.,0.,0.));
#19463=DIRECTION('center_axis',(0.,0.,-1.));
#19464=DIRECTION('ref_axis',(-1.,0.,0.));
#19465=DIRECTION('center_axis',(0.,0.,1.));
#19466=DIRECTION('ref_axis',(1.,0.,0.));
#19467=DIRECTION('center_axis',(0.,0.,1.));
#19468=DIRECTION('ref_axis',(1.,0.,0.));
#19469=DIRECTION('',(0.,0.,1.));
#19470=DIRECTION('center_axis',(-1.,0.,0.));
#19471=DIRECTION('ref_axis',(0.,1.,0.));
#19472=DIRECTION('',(0.707106781186548,0.707106781186548,8.65956056235493E-17));
#19473=DIRECTION('center_axis',(1.,0.,0.));
#19474=DIRECTION('ref_axis',(0.,0.,-1.));
#19475=DIRECTION('center_axis',(1.,0.,0.));
#19476=DIRECTION('ref_axis',(0.,0.,-1.));
#19477=DIRECTION('center_axis',(0.,0.,1.));
#19478=DIRECTION('ref_axis',(1.11022302462516E-15,-1.,0.));
#19479=DIRECTION('',(0.,0.,1.));
#19480=DIRECTION('center_axis',(0.,-1.,0.));
#19481=DIRECTION('ref_axis',(1.,0.,0.));
#19482=DIRECTION('',(0.,0.,1.));
#19483=DIRECTION('center_axis',(0.,0.,1.));
#19484=DIRECTION('ref_axis',(-1.,0.,0.));
#19485=DIRECTION('',(0.,0.,1.));
#19486=DIRECTION('center_axis',(0.,0.,1.));
#19487=DIRECTION('ref_axis',(0.,1.,0.));
#19488=DIRECTION('',(0.,0.,1.));
#19489=DIRECTION('',(0.,0.,1.));
#19490=DIRECTION('center_axis',(0.,1.,0.));
#19491=DIRECTION('ref_axis',(-1.,0.,0.));
#19492=DIRECTION('center_axis',(0.,0.,1.));
#19493=DIRECTION('ref_axis',(0.,1.,0.));
#19494=DIRECTION('center_axis',(-1.,0.,0.));
#19495=DIRECTION('ref_axis',(0.,-1.,0.));
#19496=DIRECTION('center_axis',(-1.,0.,0.));
#19497=DIRECTION('ref_axis',(0.,-1.,0.));
#19498=DIRECTION('center_axis',(0.,0.,1.));
#19499=DIRECTION('ref_axis',(-1.,0.,0.));
#19500=DIRECTION('center_axis',(0.,0.,1.));
#19501=DIRECTION('ref_axis',(-1.,0.,0.));
#19502=DIRECTION('',(0.,0.,1.));
#19503=DIRECTION('center_axis',(0.,0.,1.));
#19504=DIRECTION('ref_axis',(1.,5.55111512312577E-16,0.));
#19505=DIRECTION('center_axis',(0.,0.,1.));
#19506=DIRECTION('ref_axis',(2.22044604925031E-15,-1.,0.));
#19507=DIRECTION('center_axis',(0.,-1.,0.));
#19508=DIRECTION('ref_axis',(1.,0.,0.));
#19509=DIRECTION('',(0.,0.,1.));
#19510=DIRECTION('center_axis',(0.,0.,1.));
#19511=DIRECTION('ref_axis',(0.,1.,0.));
#19512=DIRECTION('',(0.,0.,1.));
#19513=DIRECTION('center_axis',(0.,1.,0.));
#19514=DIRECTION('ref_axis',(-1.,0.,0.));
#19515=DIRECTION('',(0.,0.,1.));
#19516=DIRECTION('center_axis',(0.,0.,1.));
#19517=DIRECTION('ref_axis',(1.,5.55111512312577E-16,0.));
#19518=DIRECTION('center_axis',(0.,0.,1.));
#19519=DIRECTION('ref_axis',(2.22044604925031E-15,-1.,0.));
#22942=CARTESIAN_POINT('',(0.,0.,0.));
#22943=CARTESIAN_POINT('Origin',(58.2244456071868,21.8438037119117,-77.));
#22944=CARTESIAN_POINT('',(58.6696447864562,21.6876074238235,-65.));
#22945=CARTESIAN_POINT('',(57.7792464279174,22.,-63.8675394171604));
#22946=CARTESIAN_POINT('Ctrl Pts',(57.7792464279174,22.,-63.8675394171605));
#22947=CARTESIAN_POINT('Ctrl Pts',(58.0193269966195,21.9157687268541,-64.0396955883018));
#22948=CARTESIAN_POINT('Ctrl Pts',(58.2665499426558,21.8290315802033,-64.2476809249266));
#22949=CARTESIAN_POINT('Ctrl Pts',(58.509255456617,21.7438793558854,-64.5516946338151));
#22950=CARTESIAN_POINT('Ctrl Pts',(58.5797344225006,21.71915210262,-64.6587247347519));
#22951=CARTESIAN_POINT('Ctrl Pts',(58.6491007720389,21.6948152061911,-64.8305933389432));
#22952=CARTESIAN_POINT('Ctrl Pts',(58.6696447864562,21.6876074238235,-64.9218325844837));
#22953=CARTESIAN_POINT('Ctrl Pts',(58.6696447864562,21.6876074238235,-65.));
#22954=CARTESIAN_POINT('',(57.7792464279174,22.,-63.));
#22955=CARTESIAN_POINT('',(57.7792464279174,22.,-77.));
#22956=CARTESIAN_POINT('',(58.6696447864562,21.6876074238235,-63.));
#22957=CARTESIAN_POINT('',(58.9671340002075,21.5832345653413,-63.));
#22958=CARTESIAN_POINT('',(58.6696447864562,21.6876074238235,-77.));
#22959=CARTESIAN_POINT('Origin',(69.,22.,-77.));
#22960=CARTESIAN_POINT('',(64.2207535720826,22.,-63.));
#22961=CARTESIAN_POINT('',(65.,22.,-63.));
#22962=CARTESIAN_POINT('',(55.7461918573286,22.,-63.));
#22963=CARTESIAN_POINT('Ctrl Pts',(57.7792464279174,22.,-63.8675394171604));
#22964=CARTESIAN_POINT('Ctrl Pts',(57.7052026398309,22.,-63.7886699029518));
#22965=CARTESIAN_POINT('Ctrl Pts',(57.6267561335641,22.,-63.716205257488));
#22966=CARTESIAN_POINT('Ctrl Pts',(57.3122246076983,22.,-63.4558552064108));
#22967=CARTESIAN_POINT('Ctrl Pts',(56.9894234086433,22.,-63.274575087265));
#22968=CARTESIAN_POINT('Ctrl Pts',(56.4120540241133,22.,-63.0659599554099));
#22969=CARTESIAN_POINT('Ctrl Pts',(56.0515769235887,22.,-63.));
#22970=CARTESIAN_POINT('Ctrl Pts',(55.7461918573286,22.,-63.));
#22971=CARTESIAN_POINT('',(53.,22.,-63.));
#22972=CARTESIAN_POINT('',(65.,22.,-63.));
#22973=CARTESIAN_POINT('',(53.,22.,-46.8343975045693));
#22974=CARTESIAN_POINT('',(53.,22.,-77.));
#22975=CARTESIAN_POINT('',(69.,22.,-41.8486611264283));
#22976=CARTESIAN_POINT('Ctrl Pts',(69.,22.,-41.8486611264284));
#22977=CARTESIAN_POINT('Ctrl Pts',(61.4497577287401,22.,-44.2291219194588));
#22978=CARTESIAN_POINT('Ctrl Pts',(53.,22.,-46.8343975045693));
#22979=CARTESIAN_POINT('',(69.,22.,-63.));
#22980=CARTESIAN_POINT('',(69.,22.,-77.));
#22981=CARTESIAN_POINT('',(66.2538081426714,22.,-63.));
#22982=CARTESIAN_POINT('',(65.,22.,-63.));
#22983=CARTESIAN_POINT('',(64.2207535720826,22.,-63.8675394171604));
#22984=CARTESIAN_POINT('Ctrl Pts',(66.2538081426714,22.,-63.));
#22985=CARTESIAN_POINT('Ctrl Pts',(65.9484230764113,22.,-63.));
#22986=CARTESIAN_POINT('Ctrl Pts',(65.5879459758867,22.,-63.0659599554099));
#22987=CARTESIAN_POINT('Ctrl Pts',(65.0105765913567,22.,-63.274575087265));
#22988=CARTESIAN_POINT('Ctrl Pts',(64.6877753923017,22.,-63.4558552064108));
#22989=CARTESIAN_POINT('Ctrl Pts',(64.3732438664359,22.,-63.716205257488));
#22990=CARTESIAN_POINT('Ctrl Pts',(64.2947973601691,22.,-63.7886699029518));
#22991=CARTESIAN_POINT('Ctrl Pts',(64.2207535720826,22.,-63.8675394171604));
#22992=CARTESIAN_POINT('',(64.2207535720826,22.,-77.));
#22993=CARTESIAN_POINT('Origin',(63.7755543928132,21.8438037119117,-77.));
#22994=CARTESIAN_POINT('',(63.3303552135438,21.6876074238235,-65.));
#22995=CARTESIAN_POINT('Ctrl Pts',(63.3303552135438,21.6876074238235,-65.));
#22996=CARTESIAN_POINT('Ctrl Pts',(63.3303552135438,21.6876074238235,-64.9218325844837));
#22997=CARTESIAN_POINT('Ctrl Pts',(63.3508992279611,21.6948152061911,-64.8305933389432));
#22998=CARTESIAN_POINT('Ctrl Pts',(63.4202655774994,21.71915210262,-64.6587247347519));
#22999=CARTESIAN_POINT('Ctrl Pts',(63.490744543383,21.7438793558854,-64.5516946338151));
#23000=CARTESIAN_POINT('Ctrl Pts',(63.7334500573442,21.8290315802033,-64.2476809249266));
#23001=CARTESIAN_POINT('Ctrl Pts',(63.9806730033805,21.9157687268541,-64.0396955883018));
#23002=CARTESIAN_POINT('Ctrl Pts',(64.2207535720826,22.,-63.8675394171604));
#23003=CARTESIAN_POINT('',(63.3303552135438,21.6876074238235,-63.));
#23004=CARTESIAN_POINT('',(63.3303552135438,21.6876074238235,-77.));
#23005=CARTESIAN_POINT('',(63.0328659997925,21.5832345653413,-63.));
#23006=CARTESIAN_POINT('Origin',(61.,25.,-77.));
#23007=CARTESIAN_POINT('',(56.95,25.,-76.5));
#23008=CARTESIAN_POINT('Origin',(61.,25.,-76.5));
#23009=CARTESIAN_POINT('',(56.95,25.,-65.));
#23010=CARTESIAN_POINT('',(56.95,25.,-77.));
#23011=CARTESIAN_POINT('Origin',(61.,25.,-65.));
#23012=CARTESIAN_POINT('Origin',(61.,25.,-63.));
#23013=CARTESIAN_POINT('Origin',(61.,25.,-65.));
#23014=CARTESIAN_POINT('Origin',(63.7755543928132,-21.8438037119117,-77.));
#23015=CARTESIAN_POINT('',(63.3303552135438,-21.6876074238235,-65.));
#23016=CARTESIAN_POINT('',(64.2207535720826,-22.,-63.8675394171604));
#23017=CARTESIAN_POINT('Ctrl Pts',(64.2207535720826,-22.,-63.8675394171605));
#23018=CARTESIAN_POINT('Ctrl Pts',(63.9806730033805,-21.9157687268541,-64.0396955883018));
#23019=CARTESIAN_POINT('Ctrl Pts',(63.7334500573442,-21.8290315802033,-64.2476809249266));
#23020=CARTESIAN_POINT('Ctrl Pts',(63.490744543383,-21.7438793558854,-64.5516946338151));
#23021=CARTESIAN_POINT('Ctrl Pts',(63.4202655774994,-21.71915210262,-64.6587247347519));
#23022=CARTESIAN_POINT('Ctrl Pts',(63.3508992279611,-21.6948152061911,-64.8305933389432));
#23023=CARTESIAN_POINT('Ctrl Pts',(63.3303552135438,-21.6876074238235,-64.9218325844837));
#23024=CARTESIAN_POINT('Ctrl Pts',(63.3303552135438,-21.6876074238235,-65.));
#23025=CARTESIAN_POINT('',(64.2207535720826,-22.,-63.));
#23026=CARTESIAN_POINT('',(64.2207535720826,-22.,-77.));
#23027=CARTESIAN_POINT('',(63.3303552135438,-21.6876074238235,-63.));
#23028=CARTESIAN_POINT('',(63.0328659997925,-21.5832345653413,-63.));
#23029=CARTESIAN_POINT('',(63.3303552135438,-21.6876074238235,-77.));
#23030=CARTESIAN_POINT('Origin',(53.,-22.,-77.));
#23031=CARTESIAN_POINT('',(57.7792464279174,-22.,-63.));
#23032=CARTESIAN_POINT('',(57.,-22.,-63.));
#23033=CARTESIAN_POINT('',(66.2538081426714,-22.,-63.));
#23034=CARTESIAN_POINT('Ctrl Pts',(64.2207535720826,-22.,-63.8675394171604));
#23035=CARTESIAN_POINT('Ctrl Pts',(64.2947973601691,-22.,-63.7886699029518));
#23036=CARTESIAN_POINT('Ctrl Pts',(64.3732438664359,-22.,-63.716205257488));
#23037=CARTESIAN_POINT('Ctrl Pts',(64.6877753923017,-22.,-63.4558552064108));
#23038=CARTESIAN_POINT('Ctrl Pts',(65.0105765913567,-22.,-63.274575087265));
#23039=CARTESIAN_POINT('Ctrl Pts',(65.5879459758867,-22.,-63.0659599554099));
#23040=CARTESIAN_POINT('Ctrl Pts',(65.9484230764113,-22.,-63.));
#23041=CARTESIAN_POINT('Ctrl Pts',(66.2538081426714,-22.,-63.));
#23042=CARTESIAN_POINT('',(69.,-22.,-63.));
#23043=CARTESIAN_POINT('',(57.,-22.,-63.));
#23044=CARTESIAN_POINT('',(69.,-22.,-41.8486611264284));
#23045=CARTESIAN_POINT('',(69.,-22.,-77.));
#23046=CARTESIAN_POINT('',(53.,-22.,-46.8343975045693));
#23047=CARTESIAN_POINT('Ctrl Pts',(53.,-22.,-46.8343975045693));
#23048=CARTESIAN_POINT('Ctrl Pts',(61.4497577287401,-22.,-44.2291219194588));
#23049=CARTESIAN_POINT('Ctrl Pts',(69.,-22.,-41.8486611264284));
#23050=CARTESIAN_POINT('',(53.,-22.,-63.));
#23051=CARTESIAN_POINT('',(53.,-22.,-77.));
#23052=CARTESIAN_POINT('',(55.7461918573286,-22.,-63.));
#23053=CARTESIAN_POINT('',(57.,-22.,-63.));
#23054=CARTESIAN_POINT('',(57.7792464279174,-22.,-63.8675394171604));
#23055=CARTESIAN_POINT('Ctrl Pts',(55.7461918573286,-22.,-63.));
#23056=CARTESIAN_POINT('Ctrl Pts',(56.0515769235887,-22.,-63.));
#23057=CARTESIAN_POINT('Ctrl Pts',(56.4120540241133,-22.,-63.0659599554099));
#23058=CARTESIAN_POINT('Ctrl Pts',(56.9894234086433,-22.,-63.274575087265));
#23059=CARTESIAN_POINT('Ctrl Pts',(57.3122246076983,-22.,-63.4558552064108));
#23060=CARTESIAN_POINT('Ctrl Pts',(57.6267561335641,-22.,-63.716205257488));
#23061=CARTESIAN_POINT('Ctrl Pts',(57.7052026398309,-22.,-63.7886699029518));
#23062=CARTESIAN_POINT('Ctrl Pts',(57.7792464279174,-22.,-63.8675394171604));
#23063=CARTESIAN_POINT('',(57.7792464279174,-22.,-77.));
#23064=CARTESIAN_POINT('Origin',(58.2244456071868,-21.8438037119117,-77.));
#23065=CARTESIAN_POINT('',(58.6696447864562,-21.6876074238235,-65.));
#23066=CARTESIAN_POINT('Ctrl Pts',(58.6696447864562,-21.6876074238235,-65.));
#23067=CARTESIAN_POINT('Ctrl Pts',(58.6696447864562,-21.6876074238235,-64.9218325844837));
#23068=CARTESIAN_POINT('Ctrl Pts',(58.6491007720389,-21.6948152061911,-64.8305933389432));
#23069=CARTESIAN_POINT('Ctrl Pts',(58.5797344225006,-21.71915210262,-64.6587247347519));
#23070=CARTESIAN_POINT('Ctrl Pts',(58.509255456617,-21.7438793558854,-64.5516946338151));
#23071=CARTESIAN_POINT('Ctrl Pts',(58.2665499426558,-21.8290315802033,-64.2476809249266));
#23072=CARTESIAN_POINT('Ctrl Pts',(58.0193269966195,-21.9157687268541,-64.0396955883018));
#23073=CARTESIAN_POINT('Ctrl Pts',(57.7792464279174,-22.,-63.8675394171605));
#23074=CARTESIAN_POINT('',(58.6696447864562,-21.6876074238235,-63.));
#23075=CARTESIAN_POINT('',(58.6696447864562,-21.6876074238235,-77.));
#23076=CARTESIAN_POINT('',(58.9671340002075,-21.5832345653413,-63.));
#23077=CARTESIAN_POINT('Origin',(61.,-25.,-77.));
#23078=CARTESIAN_POINT('',(56.95,-25.,-76.5));
#23079=CARTESIAN_POINT('Origin',(61.,-25.,-76.5));
#23080=CARTESIAN_POINT('',(56.95,-25.,-65.));
#23081=CARTESIAN_POINT('',(56.95,-25.,-77.));
#23082=CARTESIAN_POINT('Origin',(61.,-25.,-65.));
#23083=CARTESIAN_POINT('Origin',(61.,-25.,-63.));
#23084=CARTESIAN_POINT('Origin',(61.,-25.,-65.));
#23085=CARTESIAN_POINT('Origin',(61.,25.,-76.75));
#23086=CARTESIAN_POINT('',(56.45,25.,-77.));
#23087=CARTESIAN_POINT('Origin',(61.,25.,-77.));
#23088=CARTESIAN_POINT('',(56.7,25.,-76.75));
#23089=CARTESIAN_POINT('Origin',(61.,4.44089209850063E-15,-77.));
#23090=CARTESIAN_POINT('',(75.,25.,-77.));
#23091=CARTESIAN_POINT('',(69.,31.,-77.));
#23092=CARTESIAN_POINT('Origin',(69.,25.,-77.));
#23093=CARTESIAN_POINT('',(75.,-25.,-77.));
#23094=CARTESIAN_POINT('',(75.,-7.,-77.));
#23095=CARTESIAN_POINT('',(69.,-31.,-77.));
#23096=CARTESIAN_POINT('Origin',(69.,-25.,-77.));
#23097=CARTESIAN_POINT('',(53.,-31.,-77.));
#23098=CARTESIAN_POINT('',(57.,-31.,-77.));
#23099=CARTESIAN_POINT('',(47.,-25.,-77.));
#23100=CARTESIAN_POINT('Origin',(53.,-25.,-77.));
#23101=CARTESIAN_POINT('',(47.,25.,-77.));
#23102=CARTESIAN_POINT('',(47.,7.,-77.));
#23103=CARTESIAN_POINT('',(53.,31.,-77.));
#23104=CARTESIAN_POINT('Origin',(53.,25.,-77.));
#23105=CARTESIAN_POINT('',(65.,31.,-77.));
#23106=CARTESIAN_POINT('',(56.45,-25.,-77.));
#23107=CARTESIAN_POINT('Origin',(61.,-25.,-77.));
#23108=CARTESIAN_POINT('',(47.95,-1.5981640728873E-15,-77.));
#23109=CARTESIAN_POINT('Origin',(61.,0.,-77.));
#23110=CARTESIAN_POINT('Origin',(61.,-25.,-76.75));
#23111=CARTESIAN_POINT('',(56.7,-25.,-76.75));
#23112=CARTESIAN_POINT('Origin',(61.,25.,81.75));
#23113=CARTESIAN_POINT('',(56.45,25.,82.));
#23114=CARTESIAN_POINT('Origin',(61.,25.,82.));
#23115=CARTESIAN_POINT('',(56.95,25.,81.5));
#23116=CARTESIAN_POINT('',(56.7,25.,81.75));
#23117=CARTESIAN_POINT('Origin',(61.,25.,81.5));
#23118=CARTESIAN_POINT('Origin',(61.,4.44089209850063E-15,82.));
#23119=CARTESIAN_POINT('',(75.,25.,82.));
#23120=CARTESIAN_POINT('',(75.,-25.,82.));
#23121=CARTESIAN_POINT('',(75.,-7.,82.));
#23122=CARTESIAN_POINT('',(69.,31.,82.));
#23123=CARTESIAN_POINT('Origin',(69.,25.,82.));
#23124=CARTESIAN_POINT('',(53.,31.,82.));
#23125=CARTESIAN_POINT('',(65.,31.,82.));
#23126=CARTESIAN_POINT('',(47.,25.,82.));
#23127=CARTESIAN_POINT('Origin',(53.,25.,82.));
#23128=CARTESIAN_POINT('',(47.,-25.,82.));
#23129=CARTESIAN_POINT('',(47.,7.,82.));
#23130=CARTESIAN_POINT('',(53.,-31.,82.));
#23131=CARTESIAN_POINT('Origin',(53.,-25.,82.));
#23132=CARTESIAN_POINT('',(69.,-31.,82.));
#23133=CARTESIAN_POINT('',(57.,-31.,82.));
#23134=CARTESIAN_POINT('Origin',(69.,-25.,82.));
#23135=CARTESIAN_POINT('',(56.45,-25.,82.));
#23136=CARTESIAN_POINT('Origin',(61.,-25.,82.));
#23137=CARTESIAN_POINT('',(47.95,1.5981640728873E-15,82.));
#23138=CARTESIAN_POINT('Origin',(61.,0.,82.));
#23139=CARTESIAN_POINT('Origin',(61.,25.,82.));
#23140=CARTESIAN_POINT('',(56.95,25.,68.));
#23141=CARTESIAN_POINT('',(56.95,25.,82.));
#23142=CARTESIAN_POINT('Origin',(61.,25.,68.));
#23143=CARTESIAN_POINT('Origin',(61.,-25.,81.75));
#23144=CARTESIAN_POINT('',(56.95,-25.,81.5));
#23145=CARTESIAN_POINT('',(56.7,-25.,81.75));
#23146=CARTESIAN_POINT('Origin',(61.,-25.,81.5));
#23147=CARTESIAN_POINT('Origin',(61.,-25.,82.));
#23148=CARTESIAN_POINT('',(56.95,-25.,68.));
#23149=CARTESIAN_POINT('',(56.95,-25.,82.));
#23150=CARTESIAN_POINT('Origin',(61.,-25.,68.));
#23151=CARTESIAN_POINT('Origin',(68.8623677453688,0.,0.));
#23152=CARTESIAN_POINT('',(70.3988103045684,21.8767588341814,-41.0566760961604));
#23153=CARTESIAN_POINT('',(69.3999656809967,21.9899954602005,-41.7277913961831));
#23154=CARTESIAN_POINT('Ctrl Pts',(69.3999656809931,21.9899954602007,-41.7277913961841));
#23155=CARTESIAN_POINT('Ctrl Pts',(69.4678965900016,21.9865949536025,-41.7081546490098));
#23156=CARTESIAN_POINT('Ctrl Pts',(69.534827005295,21.9823737618781,-41.6848857973726));
#23157=CARTESIAN_POINT('Ctrl Pts',(69.8363491690282,21.9596786155451,-41.5614939978835));
#23158=CARTESIAN_POINT('Ctrl Pts',(70.0500315229559,21.9329167792109,-41.4208836080675));
#23159=CARTESIAN_POINT('Ctrl Pts',(70.2913558806513,21.8953193808038,-41.1842361292856));
#23160=CARTESIAN_POINT('Ctrl Pts',(70.3471478562352,21.8859334155795,-41.1220341127424));
#23161=CARTESIAN_POINT('Ctrl Pts',(70.398810304567,21.8767588341803,-41.0566760961595));
#23162=CARTESIAN_POINT('',(69.3999656809967,21.9899954602005,41.7277913961831));
#23163=CARTESIAN_POINT('Origin',(69.3999656809967,0.,9.04378927871628E-16));
#23164=CARTESIAN_POINT('',(70.3988103045684,21.8767588341814,41.0566760961604));
#23165=CARTESIAN_POINT('Ctrl Pts',(70.398810304567,21.8767588341803,41.0566760961595));
#23166=CARTESIAN_POINT('Ctrl Pts',(70.2886503403277,21.8963218164135,41.1960391538931));
#23167=CARTESIAN_POINT('Ctrl Pts',(70.1605038308314,21.9167166021157,41.3200714701435));
#23168=CARTESIAN_POINT('Ctrl Pts',(69.8499581892739,21.9564850241577,41.5472005422254));
#23169=CARTESIAN_POINT('Ctrl Pts',(69.6655971081557,21.9746882921927,41.6417814905459));
#23170=CARTESIAN_POINT('Ctrl Pts',(69.4462977513165,21.9875746254245,41.7139399145121));
#23171=CARTESIAN_POINT('Ctrl Pts',(69.4231883393022,21.9888329731391,41.7210784362578));
#23172=CARTESIAN_POINT('Ctrl Pts',(69.3999656809966,21.9899954602005,41.7277913961831));
#23173=CARTESIAN_POINT('Origin',(70.3988103045635,0.,8.91992201499275E-16));
#23174=CARTESIAN_POINT('Origin',(59.25,0.,0.));
#23175=CARTESIAN_POINT('Ctrl Pts',(69.3999656809967,21.9899954602005,-41.7277913961831));
#23176=CARTESIAN_POINT('Ctrl Pts',(69.2669412328493,21.9966544394525,-41.7662446937235));
#23177=CARTESIAN_POINT('Ctrl Pts',(69.1335296058873,22.,-41.8065615513282));
#23178=CARTESIAN_POINT('Ctrl Pts',(69.,22.,-41.8486611264283));
#23179=CARTESIAN_POINT('',(48.5,20.6143782776615,-48.8267079396664));
#23180=CARTESIAN_POINT('Ctrl Pts',(53.,22.,-46.8343975045693));
#23181=CARTESIAN_POINT('Ctrl Pts',(52.220819689021,22.,-47.0746386458849));
#23182=CARTESIAN_POINT('Ctrl Pts',(51.4345269237376,21.8835425868198,-47.3718185033061));
#23183=CARTESIAN_POINT('Ctrl Pts',(49.8969249897714,21.4203044222019,-48.0534285948251));
#23184=CARTESIAN_POINT('Ctrl Pts',(49.1505318652661,21.0569585581973,-48.4427922865552));
#23185=CARTESIAN_POINT('Ctrl Pts',(48.5,20.6143782776615,-48.8267079396664));
#23186=CARTESIAN_POINT('',(48.5,20.6143782776615,48.8267079396664));
#23187=CARTESIAN_POINT('Origin',(48.5,0.,0.));
#23188=CARTESIAN_POINT('',(53.,22.,46.8343975045693));
#23189=CARTESIAN_POINT('Ctrl Pts',(48.5,20.6143782776615,48.8267079396664));
#23190=CARTESIAN_POINT('Ctrl Pts',(49.1505318652661,21.0569585581973,48.4427922865552));
#23191=CARTESIAN_POINT('Ctrl Pts',(49.8969249897714,21.4203044222019,48.0534285948251));
#23192=CARTESIAN_POINT('Ctrl Pts',(51.4345269237376,21.8835425868198,47.3718185033061));
#23193=CARTESIAN_POINT('Ctrl Pts',(52.220819689021,22.,47.0746386458849));
#23194=CARTESIAN_POINT('Ctrl Pts',(53.,22.,46.8343975045693));
#23195=CARTESIAN_POINT('',(69.,22.,41.8486611264283));
#23196=CARTESIAN_POINT('Ctrl Pts',(53.,22.,46.8343975045693));
#23197=CARTESIAN_POINT('Ctrl Pts',(61.4497577287401,22.,44.2291219194588));
#23198=CARTESIAN_POINT('Ctrl Pts',(69.,22.,41.8486611264284));
#23199=CARTESIAN_POINT('Ctrl Pts',(69.,22.,41.8486611264283));
#23200=CARTESIAN_POINT('Ctrl Pts',(69.1335306008183,22.,41.8065612376436));
#23201=CARTESIAN_POINT('Ctrl Pts',(69.266941620321,21.9966544200563,41.7662445817172));
#23202=CARTESIAN_POINT('Ctrl Pts',(69.3999656809966,21.9899954602005,41.7277913961831));
#23203=CARTESIAN_POINT('Origin',(68.8623677453688,0.,0.));
#23204=CARTESIAN_POINT('',(70.3988103045684,-21.8767588341814,41.0566760961604));
#23205=CARTESIAN_POINT('',(69.3999656809967,-21.9899954602005,41.7277913961831));
#23206=CARTESIAN_POINT('Ctrl Pts',(69.3999656809931,-21.9899954602007,41.7277913961841));
#23207=CARTESIAN_POINT('Ctrl Pts',(69.4678965900016,-21.9865949536025,41.7081546490098));
#23208=CARTESIAN_POINT('Ctrl Pts',(69.534827005295,-21.9823737618781,41.6848857973726));
#23209=CARTESIAN_POINT('Ctrl Pts',(69.8363491690282,-21.9596786155451,41.5614939978835));
#23210=CARTESIAN_POINT('Ctrl Pts',(70.0500315229559,-21.9329167792109,41.4208836080676));
#23211=CARTESIAN_POINT('Ctrl Pts',(70.2913558806513,-21.8953193808038,41.1842361292856));
#23212=CARTESIAN_POINT('Ctrl Pts',(70.3471478562352,-21.8859334155794,41.1220341127424));
#23213=CARTESIAN_POINT('Ctrl Pts',(70.398810304567,-21.8767588341803,41.0566760961595));
#23214=CARTESIAN_POINT('',(69.3999656809967,-21.9899954602005,-41.7277913961831));
#23215=CARTESIAN_POINT('Origin',(69.3999656809967,0.,-7.2204335534144E-15));
#23216=CARTESIAN_POINT('',(70.3988103045683,-21.8767588341814,-41.0566760961604));
#23217=CARTESIAN_POINT('Ctrl Pts',(70.398810304567,-21.8767588341803,-41.0566760961595));
#23218=CARTESIAN_POINT('Ctrl Pts',(70.2886503403277,-21.8963218164135,-41.1960391538931));
#23219=CARTESIAN_POINT('Ctrl Pts',(70.1605038308314,-21.9167166021156,-41.3200714701435));
#23220=CARTESIAN_POINT('Ctrl Pts',(69.8499581892738,-21.9564850241576,-41.5472005422254));
#23221=CARTESIAN_POINT('Ctrl Pts',(69.6655971081557,-21.9746882921927,-41.6417814905459));
#23222=CARTESIAN_POINT('Ctrl Pts',(69.4462977513165,-21.9875746254244,-41.7139399145121));
#23223=CARTESIAN_POINT('Ctrl Pts',(69.4231883393022,-21.988832973139,-41.7210784362578));
#23224=CARTESIAN_POINT('Ctrl Pts',(69.3999656809966,-21.9899954602005,-41.7277913961831));
#23225=CARTESIAN_POINT('',(70.3988103045635,-46.5214276345238,-5.69723174443847E-15));
#23226=CARTESIAN_POINT('Origin',(70.3988103045635,0.,-7.12153968054809E-15));
#23227=CARTESIAN_POINT('Origin',(70.3988103045635,0.,-7.12153968054809E-15));
#23228=CARTESIAN_POINT('Origin',(59.25,0.,0.));
#23229=CARTESIAN_POINT('',(69.,-22.,41.8486611264284));
#23230=CARTESIAN_POINT('Ctrl Pts',(69.3999656809967,-21.9899954602005,41.7277913961831));
#23231=CARTESIAN_POINT('Ctrl Pts',(69.2669412328493,-21.9966544394524,41.7662446937235));
#23232=CARTESIAN_POINT('Ctrl Pts',(69.1335296058873,-22.,41.8065615513282));
#23233=CARTESIAN_POINT('Ctrl Pts',(69.,-22.,41.8486611264284));
#23234=CARTESIAN_POINT('',(53.,-22.,46.8343975045693));
#23235=CARTESIAN_POINT('Ctrl Pts',(69.,-22.,41.8486611264284));
#23236=CARTESIAN_POINT('Ctrl Pts',(61.4497577287401,-22.,44.2291219194588));
#23237=CARTESIAN_POINT('Ctrl Pts',(53.,-22.,46.8343975045693));
#23238=CARTESIAN_POINT('',(48.5,-20.6143782776615,48.8267079396664));
#23239=CARTESIAN_POINT('Ctrl Pts',(53.,-22.,46.8343975045693));
#23240=CARTESIAN_POINT('Ctrl Pts',(52.220819689021,-22.,47.0746386458849));
#23241=CARTESIAN_POINT('Ctrl Pts',(51.4345269237375,-21.8835425868198,47.3718185033061));
#23242=CARTESIAN_POINT('Ctrl Pts',(49.8969249897714,-21.4203044222019,48.0534285948251));
#23243=CARTESIAN_POINT('Ctrl Pts',(49.1505318652661,-21.0569585581973,48.4427922865552));
#23244=CARTESIAN_POINT('Ctrl Pts',(48.5,-20.6143782776615,48.8267079396664));
#23245=CARTESIAN_POINT('',(48.5,-20.6143782776615,-48.8267079396664));
#23246=CARTESIAN_POINT('Origin',(48.5,0.,0.));
#23247=CARTESIAN_POINT('Ctrl Pts',(48.5,-20.6143782776615,-48.8267079396664));
#23248=CARTESIAN_POINT('Ctrl Pts',(49.1505318652661,-21.0569585581973,-48.4427922865552));
#23249=CARTESIAN_POINT('Ctrl Pts',(49.8969249897714,-21.4203044222019,-48.0534285948251));
#23250=CARTESIAN_POINT('Ctrl Pts',(51.4345269237375,-21.8835425868198,-47.3718185033061));
#23251=CARTESIAN_POINT('Ctrl Pts',(52.220819689021,-22.,-47.0746386458849));
#23252=CARTESIAN_POINT('Ctrl Pts',(53.,-22.,-46.8343975045693));
#23253=CARTESIAN_POINT('Ctrl Pts',(69.,-22.,-41.8486611264283));
#23254=CARTESIAN_POINT('Ctrl Pts',(69.1335306008184,-22.,-41.8065612376436));
#23255=CARTESIAN_POINT('Ctrl Pts',(69.266941620321,-21.9966544200563,-41.7662445817172));
#23256=CARTESIAN_POINT('Ctrl Pts',(69.3999656809967,-21.9899954602005,-41.7277913961831));
#23257=CARTESIAN_POINT('Origin',(78.,0.,0.));
#23258=CARTESIAN_POINT('',(80.,-4.19758713816547E-15,34.2759001296373));
#23259=CARTESIAN_POINT('Origin',(80.,0.,0.));
#23260=CARTESIAN_POINT('',(79.5364425591947,-4.35438709334811E-15,35.5562689289663));
#23261=CARTESIAN_POINT('Origin',(78.,-4.19758713816547E-15,34.2759001296373));
#23262=CARTESIAN_POINT('',(79.5364425591948,-35.5562689289663,-4.35438709334811E-15));
#23263=CARTESIAN_POINT('Origin',(79.5364425591947,0.,-5.44298386668513E-15));
#23264=CARTESIAN_POINT('Origin',(79.5364425591947,0.,-5.44298386668513E-15));
#23265=CARTESIAN_POINT('Origin',(75.,0.,0.));
#23266=CARTESIAN_POINT('',(75.,-41.,-5.02105187650415E-15));
#23267=CARTESIAN_POINT('',(77.,-14.,-35.9716555081915));
#23268=CARTESIAN_POINT('Ctrl Pts',(70.398810304567,-21.8767588341803,-41.0566760961595));
#23269=CARTESIAN_POINT('Ctrl Pts',(71.2727530473023,-21.7215579273257,-39.9510536156882));
#23270=CARTESIAN_POINT('Ctrl Pts',(72.1553913142385,-21.4169490490281,-38.9085591876444));
#23271=CARTESIAN_POINT('Ctrl Pts',(73.0068003967573,-20.9242725668871,-38.0135049004133));
#23272=CARTESIAN_POINT('Ctrl Pts',(73.6552875413432,-20.5490189177681,-37.3317748004022));
#23273=CARTESIAN_POINT('Ctrl Pts',(74.3605604649236,-20.0126010939214,-36.6628462695613));
#23274=CARTESIAN_POINT('Ctrl Pts',(75.2978777322535,-18.9556514474071,-35.9519067932131));
#23275=CARTESIAN_POINT('Ctrl Pts',(75.5909608136772,-18.5615213463442,-35.7620681117759));
#23276=CARTESIAN_POINT('Ctrl Pts',(76.10601454772,-17.7084765949661,-35.5027149353752));
#23277=CARTESIAN_POINT('Ctrl Pts',(76.3278529636206,-17.2494659834457,-35.4332534860856));
#23278=CARTESIAN_POINT('Ctrl Pts',(76.6706196605434,-16.3224653535192,-35.4171046265844));
#23279=CARTESIAN_POINT('Ctrl Pts',(76.7982138286546,-15.8499176073548,-35.4643373367294));
#23280=CARTESIAN_POINT('Ctrl Pts',(76.9611527928263,-14.9146287542956,-35.6556385052494));
#23281=CARTESIAN_POINT('Ctrl Pts',(77.,-14.4521831933392,-35.795667925265));
#23282=CARTESIAN_POINT('Ctrl Pts',(77.,-14.,-35.9716555081914));
#23283=CARTESIAN_POINT('',(77.,14.,-35.9716555081914));
#23284=CARTESIAN_POINT('Origin',(77.,0.,0.));
#23285=CARTESIAN_POINT('Ctrl Pts',(77.,14.,-35.9716555081914));
#23286=CARTESIAN_POINT('Ctrl Pts',(77.,14.4521831933392,-35.795667925265));
#23287=CARTESIAN_POINT('Ctrl Pts',(76.9611527928263,14.9146287542956,-35.6556385052494));
#23288=CARTESIAN_POINT('Ctrl Pts',(76.7982138286546,15.8499176073548,-35.4643373367294));
#23289=CARTESIAN_POINT('Ctrl Pts',(76.6706196605434,16.3224653535192,-35.4171046265844));
#23290=CARTESIAN_POINT('Ctrl Pts',(76.3278529636206,17.2494659834456,-35.4332534860856));
#23291=CARTESIAN_POINT('Ctrl Pts',(76.10601454772,17.7084765949661,-35.5027149353752));
#23292=CARTESIAN_POINT('Ctrl Pts',(75.5909608136772,18.5615213463443,-35.7620681117759));
#23293=CARTESIAN_POINT('Ctrl Pts',(75.2978777322535,18.9556514474071,-35.9519067932131));
#23294=CARTESIAN_POINT('Ctrl Pts',(74.3605604649237,20.0126010939214,-36.6628462695613));
#23295=CARTESIAN_POINT('Ctrl Pts',(73.6552875413432,20.5490189177681,-37.3317748004022));
#23296=CARTESIAN_POINT('Ctrl Pts',(72.1553913142392,21.4169490490277,-38.9085591876437));
#23297=CARTESIAN_POINT('Ctrl Pts',(71.2727530473009,21.7215579273259,-39.9510536156899));
#23298=CARTESIAN_POINT('Ctrl Pts',(70.398810304567,21.8767588341803,-41.0566760961595));
#23299=CARTESIAN_POINT('',(77.,14.,35.9716555081914));
#23300=CARTESIAN_POINT('Ctrl Pts',(70.398810304567,21.8767588341803,41.0566760961595));
#23301=CARTESIAN_POINT('Ctrl Pts',(71.2727530473009,21.7215579273259,39.9510536156899));
#23302=CARTESIAN_POINT('Ctrl Pts',(72.1553913142392,21.4169490490277,38.9085591876437));
#23303=CARTESIAN_POINT('Ctrl Pts',(73.6552875413432,20.5490189177681,37.3317748004022));
#23304=CARTESIAN_POINT('Ctrl Pts',(74.3605604649237,20.0126010939214,36.6628462695613));
#23305=CARTESIAN_POINT('Ctrl Pts',(75.2978777322535,18.9556514474071,35.9519067932131));
#23306=CARTESIAN_POINT('Ctrl Pts',(75.5909608136772,18.5615213463442,35.7620681117759));
#23307=CARTESIAN_POINT('Ctrl Pts',(76.10601454772,17.7084765949661,35.5027149353752));
#23308=CARTESIAN_POINT('Ctrl Pts',(76.3278529636206,17.2494659834457,35.4332534860856));
#23309=CARTESIAN_POINT('Ctrl Pts',(76.6706196605434,16.3224653535192,35.4171046265844));
#23310=CARTESIAN_POINT('Ctrl Pts',(76.7982138286546,15.8499176073548,35.4643373367294));
#23311=CARTESIAN_POINT('Ctrl Pts',(76.9611527928263,14.9146287542956,35.6556385052494));
#23312=CARTESIAN_POINT('Ctrl Pts',(77.,14.4521831933392,35.795667925265));
#23313=CARTESIAN_POINT('Ctrl Pts',(77.,14.,35.9716555081914));
#23314=CARTESIAN_POINT('',(77.,-14.,35.9716555081915));
#23315=CARTESIAN_POINT('Origin',(77.,0.,0.));
#23316=CARTESIAN_POINT('Ctrl Pts',(77.,-14.,35.9716555081914));
#23317=CARTESIAN_POINT('Ctrl Pts',(77.,-14.4521831941371,35.7956679249545));
#23318=CARTESIAN_POINT('Ctrl Pts',(76.9611527928323,-14.9146287542614,35.6556385052564));
#23319=CARTESIAN_POINT('Ctrl Pts',(76.7982138286546,-15.8499176073548,35.4643373367294));
#23320=CARTESIAN_POINT('Ctrl Pts',(76.6706196605434,-16.3224653535192,35.4171046265844));
#23321=CARTESIAN_POINT('Ctrl Pts',(76.3278529636206,-17.2494659834457,35.4332534860856));
#23322=CARTESIAN_POINT('Ctrl Pts',(76.10601454772,-17.7084765949661,35.5027149353752));
#23323=CARTESIAN_POINT('Ctrl Pts',(75.5909608136772,-18.5615213463442,35.7620681117759));
#23324=CARTESIAN_POINT('Ctrl Pts',(75.2978777322535,-18.9556514474071,35.9519067932131));
#23325=CARTESIAN_POINT('Ctrl Pts',(74.3605604649236,-20.0126010939214,36.6628462695613));
#23326=CARTESIAN_POINT('Ctrl Pts',(73.6552875413432,-20.5490189177681,37.3317748004022));
#23327=CARTESIAN_POINT('Ctrl Pts',(73.0068003967573,-20.9242725668871,38.0135049004133));
#23328=CARTESIAN_POINT('Ctrl Pts',(72.1553913142392,-21.4169490490277,38.9085591876437));
#23329=CARTESIAN_POINT('Ctrl Pts',(71.2727530473009,-21.7215579273259,39.9510536156899));
#23330=CARTESIAN_POINT('Ctrl Pts',(70.398810304567,-21.8767588341803,41.0566760961595));
#23331=CARTESIAN_POINT('Origin',(80.,0.,0.));
#23332=CARTESIAN_POINT('',(80.,2.,-8.));
#23333=CARTESIAN_POINT('',(80.,1.99999999999999,-33.));
#23334=CARTESIAN_POINT('',(80.,2.,-16.5));
#23335=CARTESIAN_POINT('',(80.,-2.00000000000001,-33.));
#23336=CARTESIAN_POINT('',(80.,-1.,-33.));
#23337=CARTESIAN_POINT('',(80.,-2.,-8.));
#23338=CARTESIAN_POINT('',(80.,-2.,-4.));
#23339=CARTESIAN_POINT('',(80.,0.999999999999999,-8.));
#23340=CARTESIAN_POINT('',(80.,5.92820323027551,5.73205080756888));
#23341=CARTESIAN_POINT('',(80.,27.5788383248865,18.2320508075689));
#23342=CARTESIAN_POINT('',(80.,13.2894191624432,9.98205080756887));
#23343=CARTESIAN_POINT('',(80.,29.5788383248865,14.7679491924311));
#23344=CARTESIAN_POINT('',(80.,29.0788383248865,15.6339745962156));
#23345=CARTESIAN_POINT('',(80.,7.92820323027551,2.26794919243112));
#23346=CARTESIAN_POINT('',(80.,4.46410161513776,0.267949192431122));
#23347=CARTESIAN_POINT('',(80.,6.42820323027551,4.86602540378444));
#23348=CARTESIAN_POINT('',(80.,-2.,8.));
#23349=CARTESIAN_POINT('',(80.,-2.,33.));
#23350=CARTESIAN_POINT('',(80.,-2.,16.5));
#23351=CARTESIAN_POINT('',(80.,2.,33.));
#23352=CARTESIAN_POINT('',(80.,1.,33.));
#23353=CARTESIAN_POINT('',(80.,2.,8.));
#23354=CARTESIAN_POINT('',(80.,2.,4.));
#23355=CARTESIAN_POINT('',(80.,-1.,8.));
#23356=CARTESIAN_POINT('',(80.,-7.92820323027551,2.26794919243112));
#23357=CARTESIAN_POINT('',(80.,-29.5788383248865,14.7679491924311));
#23358=CARTESIAN_POINT('',(80.,-15.2894191624432,6.51794919243112));
#23359=CARTESIAN_POINT('',(80.,-27.5788383248865,18.2320508075689));
#23360=CARTESIAN_POINT('',(80.,-28.0788383248865,17.3660254037844));
#23361=CARTESIAN_POINT('',(80.,-5.92820323027551,5.73205080756888));
#23362=CARTESIAN_POINT('',(80.,-2.46410161513775,3.73205080756888));
#23363=CARTESIAN_POINT('',(80.,-7.42820323027551,3.13397459621556));
#23364=CARTESIAN_POINT('',(80.,-5.92820323027551,-5.73205080756888));
#23365=CARTESIAN_POINT('',(80.,-27.5788383248865,-18.2320508075689));
#23366=CARTESIAN_POINT('',(80.,-13.2894191624432,-9.98205080756888));
#23367=CARTESIAN_POINT('',(80.,-29.5788383248865,-14.7679491924311));
#23368=CARTESIAN_POINT('',(80.,-29.0788383248865,-15.6339745962156));
#23369=CARTESIAN_POINT('',(80.,-7.92820323027551,-2.26794919243112));
#23370=CARTESIAN_POINT('',(80.,-4.46410161513775,-0.267949192431123));
#23371=CARTESIAN_POINT('',(80.,-6.42820323027551,-4.86602540378444));
#23372=CARTESIAN_POINT('',(80.,7.92820323027551,-2.26794919243113));
#23373=CARTESIAN_POINT('',(80.,29.5788383248865,-14.7679491924311));
#23374=CARTESIAN_POINT('',(80.,15.2894191624432,-6.51794919243113));
#23375=CARTESIAN_POINT('',(80.,27.5788383248865,-18.2320508075689));
#23376=CARTESIAN_POINT('',(80.,28.0788383248865,-17.3660254037845));
#23377=CARTESIAN_POINT('',(80.,5.92820323027551,-5.73205080756888));
#23378=CARTESIAN_POINT('',(80.,2.46410161513775,-3.73205080756888));
#23379=CARTESIAN_POINT('',(80.,7.42820323027551,-3.13397459621557));
#23380=CARTESIAN_POINT('Origin',(46.5,0.,-2.20309881449055E-15));
#23381=CARTESIAN_POINT('',(48.5,-29.0466953015038,65.0006740405344));
#23382=CARTESIAN_POINT('',(48.0857864376269,-30.6065287460451,65.6281854386855));
#23383=CARTESIAN_POINT('Ctrl Pts',(48.0857864376269,-30.6065287460451,65.6281854386855));
#23384=CARTESIAN_POINT('Ctrl Pts',(48.1301492537468,-30.5806858219106,65.576544441517));
#23385=CARTESIAN_POINT('Ctrl Pts',(48.1707278411709,-30.5469525825928,65.5268107752811));
#23386=CARTESIAN_POINT('Ctrl Pts',(48.2441371413255,-30.4644482587098,65.4324498012713));
#23387=CARTESIAN_POINT('Ctrl Pts',(48.2762461582976,-30.4166263879609,65.3887900387193));
#23388=CARTESIAN_POINT('Ctrl Pts',(48.3631644375932,-30.2517748834464,65.2649170060744));
#23389=CARTESIAN_POINT('Ctrl Pts',(48.4031257978626,-30.1193145924239,65.1990939013729));
#23390=CARTESIAN_POINT('Ctrl Pts',(48.4773089651312,-29.7481720100829,65.0666632800059));
#23391=CARTESIAN_POINT('Ctrl Pts',(48.4999999982949,-29.4453272025579,65.007596110854));
#23392=CARTESIAN_POINT('Ctrl Pts',(48.5,-29.0466953013294,65.0006740505758));
#23393=CARTESIAN_POINT('',(48.0857864376272,-31.3127256445526,-65.2941922269196));
#23394=CARTESIAN_POINT('Origin',(48.0857864376269,0.,-2.20309881449055E-15));
#23395=CARTESIAN_POINT('',(48.2311293323885,-31.4232291377153,-64.9999999933255));
#23396=CARTESIAN_POINT('Ctrl Pts',(48.2311293323885,-31.4232291377153,-64.9999999933255));
#23397=CARTESIAN_POINT('Ctrl Pts',(48.1867097281574,-31.3902501884761,-65.1012175444252));
#23398=CARTESIAN_POINT('Ctrl Pts',(48.1379693104345,-31.3533479994135,-65.1994072998738));
#23399=CARTESIAN_POINT('Ctrl Pts',(48.0857864376269,-31.3127256445523,-65.29419222692));
#23400=CARTESIAN_POINT('',(48.5,-31.2619954337637,-63.9647228889383));
#23401=CARTESIAN_POINT('Ctrl Pts',(48.5,-31.2619954300771,-63.9647228854569));
#23402=CARTESIAN_POINT('Ctrl Pts',(48.5,-31.3066103800828,-64.0246074793082));
#23403=CARTESIAN_POINT('Ctrl Pts',(48.4959556515835,-31.3454934513646,-64.0880064784246));
#23404=CARTESIAN_POINT('Ctrl Pts',(48.4796166024191,-31.409284557683,-64.2199289334738));
#23405=CARTESIAN_POINT('Ctrl Pts',(48.4676779476615,-31.4339507060007,-64.2871111751952));
#23406=CARTESIAN_POINT('Ctrl Pts',(48.420825382814,-31.4874720705551,-64.4950891861979));
#23407=CARTESIAN_POINT('Ctrl Pts',(48.3762987971587,-31.4934261407582,-64.6350319244059));
#23408=CARTESIAN_POINT('Ctrl Pts',(48.2959416031664,-31.4655323782762,-64.8476351547665));
#23409=CARTESIAN_POINT('Ctrl Pts',(48.2645571018583,-31.4480472944176,-64.9238291895505));
#23410=CARTESIAN_POINT('Ctrl Pts',(48.2311293323885,-31.4232291377153,-64.9999999933256));
#23411=CARTESIAN_POINT('Origin',(48.5,0.,-2.20309881449055E-15));
#23412=CARTESIAN_POINT('Origin',(48.5,53.,0.));
#23413=CARTESIAN_POINT('',(48.5,-28.9686269665969,-63.));
#23414=CARTESIAN_POINT('Ctrl Pts',(48.5,-31.2619954330609,-63.964722889462));
#23415=CARTESIAN_POINT('Ctrl Pts',(48.5,-31.1786502720937,-63.8528525155057));
#23416=CARTESIAN_POINT('Ctrl Pts',(48.5,-31.0821687424774,-63.7502960288675));
#23417=CARTESIAN_POINT('Ctrl Pts',(48.5,-30.7662183987535,-63.4685459818617));
#23418=CARTESIAN_POINT('Ctrl Pts',(48.5,-30.4573223491148,-63.2950310532685));
#23419=CARTESIAN_POINT('Ctrl Pts',(48.5,-29.8155012575532,-63.0638354527098));
#23420=CARTESIAN_POINT('Ctrl Pts',(48.5,-29.3555738612142,-63.));
#23421=CARTESIAN_POINT('Ctrl Pts',(48.5,-28.9686269665969,-63.));
#23422=CARTESIAN_POINT('',(48.5,-20.6143782776615,-63.));
#23423=CARTESIAN_POINT('',(48.5,26.5,-63.));
#23424=CARTESIAN_POINT('',(48.5,-20.6143782776615,-77.));
#23425=CARTESIAN_POINT('',(48.5,-20.6143782776615,65.));
#23426=CARTESIAN_POINT('',(48.5,-20.6143782776615,-77.));
#23427=CARTESIAN_POINT('',(48.5,-28.9686269665969,65.));
#23428=CARTESIAN_POINT('',(48.5,26.5,65.));
#23429=CARTESIAN_POINT('Ctrl Pts',(48.5,-28.9686269665969,65.));
#23430=CARTESIAN_POINT('Ctrl Pts',(48.5,-28.9943212164188,65.));
#23431=CARTESIAN_POINT('Ctrl Pts',(48.5,-29.0203628803793,65.0002168001558));
#23432=CARTESIAN_POINT('Ctrl Pts',(48.5,-29.0466953013294,65.0006740505758));
#23433=CARTESIAN_POINT('',(48.5,-62.,4.50000000000001));
#23434=CARTESIAN_POINT('Origin',(48.5,-62.,7.59281015471359E-15));
#23435=CARTESIAN_POINT('',(48.5,-31.,58.1935750346352));
#23436=CARTESIAN_POINT('Origin',(48.5,-31.,53.6935750346352));
#23437=CARTESIAN_POINT('',(48.5,-31.,-49.1935750346352));
#23438=CARTESIAN_POINT('Origin',(48.5,-31.,-53.6935750346352));
#23439=CARTESIAN_POINT('Origin',(46.6715728752538,0.,0.));
#23440=CARTESIAN_POINT('',(46.671572875469,-29.8356437966493,66.6245777415471));
#23441=CARTESIAN_POINT('Ctrl Pts',(46.6715728756007,-29.8356437965537,66.62457774159));
#23442=CARTESIAN_POINT('Ctrl Pts',(46.9003594149229,-30.0980676345434,66.5070597861704));
#23443=CARTESIAN_POINT('Ctrl Pts',(47.1258706110947,-30.2962111663502,66.3731410562788));
#23444=CARTESIAN_POINT('Ctrl Pts',(47.5020219686064,-30.5347787801062,66.1177462694265));
#23445=CARTESIAN_POINT('Ctrl Pts',(47.6577886183648,-30.5990942737804,66.0001438773577));
#23446=CARTESIAN_POINT('Ctrl Pts',(47.8979638703951,-30.6386169314764,65.801001256245));
#23447=CARTESIAN_POINT('Ctrl Pts',(47.9949018863232,-30.6355802321398,65.7149190292199));
#23448=CARTESIAN_POINT('Ctrl Pts',(48.0857864376269,-30.6065287460451,65.6281854386855));
#23449=CARTESIAN_POINT('',(46.6715728756007,-73.,-8.93992163377568E-15));
#23450=CARTESIAN_POINT('Origin',(46.6715728752538,0.,0.));
#23451=CARTESIAN_POINT('',(46.6715728752538,-29.8939769234005,-66.5984244836407));
#23452=CARTESIAN_POINT('Origin',(46.6715728752538,0.,0.));
#23453=CARTESIAN_POINT('Ctrl Pts',(48.0857864376272,-31.3127256445525,-65.2941922269195));
#23454=CARTESIAN_POINT('Ctrl Pts',(47.8770411481129,-31.1502254836754,-65.6036293796078));
#23455=CARTESIAN_POINT('Ctrl Pts',(47.6239041583091,-30.9374332353599,-65.8819860357444));
#23456=CARTESIAN_POINT('Ctrl Pts',(47.1265432809023,-30.4403912323438,-66.3084804710889));
#23457=CARTESIAN_POINT('Ctrl Pts',(46.8987540346771,-30.187746067397,-66.4665605832628));
#23458=CARTESIAN_POINT('Ctrl Pts',(46.6715728752538,-29.8939769234005,-66.5984244836407));
#23459=CARTESIAN_POINT('Origin',(43.5,0.,0.));
#23460=CARTESIAN_POINT('',(46.0618680733842,-28.9827534908495,67.0000000003308));
#23461=CARTESIAN_POINT('Ctrl Pts',(46.6715728756007,-29.8356437965537,66.62457774159));
#23462=CARTESIAN_POINT('Ctrl Pts',(46.4403768088297,-29.570456170775,66.7433333691705));
#23463=CARTESIAN_POINT('Ctrl Pts',(46.235774905439,-29.2857068488205,66.8689489186728));
#23464=CARTESIAN_POINT('Ctrl Pts',(46.0618680734383,-28.9827534909439,67.0000000006207));
#23465=CARTESIAN_POINT('',(45.,-25.,68.585712797929));
#23466=CARTESIAN_POINT('Ctrl Pts',(46.0618680734383,-28.9827534909439,67.0000000006207));
#23467=CARTESIAN_POINT('Ctrl Pts',(45.9012005717238,-28.7028636293842,67.1210743119957));
#23468=CARTESIAN_POINT('Ctrl Pts',(45.757046826217,-28.4123616493805,67.244642097791));
#23469=CARTESIAN_POINT('Ctrl Pts',(45.2085080184809,-27.1145210836178,67.7862582857373));
#23470=CARTESIAN_POINT('Ctrl Pts',(45.,-26.0264488036591,68.211564611016));
#23471=CARTESIAN_POINT('Ctrl Pts',(45.,-25.,68.585712797929));
#23472=CARTESIAN_POINT('',(45.,25.,68.585712797929));
#23473=CARTESIAN_POINT('Origin',(45.,0.,0.));
#23474=CARTESIAN_POINT('',(46.0618680733842,28.9827534908495,67.0000000003308));
#23475=CARTESIAN_POINT('Ctrl Pts',(45.,25.,68.585712797929));
#23476=CARTESIAN_POINT('Ctrl Pts',(45.,26.0264488036591,68.211564611016));
#23477=CARTESIAN_POINT('Ctrl Pts',(45.2085080184809,27.1145210836178,67.7862582857373));
#23478=CARTESIAN_POINT('Ctrl Pts',(45.757046826217,28.4123616493805,67.244642097791));
#23479=CARTESIAN_POINT('Ctrl Pts',(45.9012005717238,28.7028636293842,67.1210743119957));
#23480=CARTESIAN_POINT('Ctrl Pts',(46.0618680734383,28.9827534909439,67.0000000006207));
#23481=CARTESIAN_POINT('',(46.6715728753143,29.8356437962946,66.624577741706));
#23482=CARTESIAN_POINT('Ctrl Pts',(46.0618680734383,28.9827534909439,67.0000000006207));
#23483=CARTESIAN_POINT('Ctrl Pts',(46.2356286911114,29.2854521370245,66.8690591014966));
#23484=CARTESIAN_POINT('Ctrl Pts',(46.4402143281585,29.5702698013771,66.7434168286244));
#23485=CARTESIAN_POINT('Ctrl Pts',(46.6715728753514,29.8356437962676,66.6245777417181));
#23486=CARTESIAN_POINT('',(46.6715728752538,29.8939769234005,-66.5984244836407));
#23487=CARTESIAN_POINT('Origin',(46.6715728752538,0.,0.));
#23488=CARTESIAN_POINT('',(45.,25.,-68.585712797929));
#23489=CARTESIAN_POINT('Ctrl Pts',(46.6715728752538,29.8939769234005,-66.5984244836407));
#23490=CARTESIAN_POINT('Ctrl Pts',(46.2545757421566,29.3547557522879,-66.8404642221305));
#23491=CARTESIAN_POINT('Ctrl Pts',(45.9004614465488,28.751680051953,-67.1030373856642));
#23492=CARTESIAN_POINT('Ctrl Pts',(45.2085080184809,27.1145210836178,-67.7862582857373));
#23493=CARTESIAN_POINT('Ctrl Pts',(45.,26.0264488036591,-68.211564611016));
#23494=CARTESIAN_POINT('Ctrl Pts',(45.,25.,-68.585712797929));
#23495=CARTESIAN_POINT('',(45.,-25.,-68.585712797929));
#23496=CARTESIAN_POINT('Origin',(45.,0.,0.));
#23497=CARTESIAN_POINT('Ctrl Pts',(45.,-25.,-68.585712797929));
#23498=CARTESIAN_POINT('Ctrl Pts',(45.,-26.0264488036591,-68.211564611016));
#23499=CARTESIAN_POINT('Ctrl Pts',(45.2085080184809,-27.1145210836178,-67.7862582857373));
#23500=CARTESIAN_POINT('Ctrl Pts',(45.9004614465488,-28.751680051953,-67.1030373856642));
#23501=CARTESIAN_POINT('Ctrl Pts',(46.2545757421565,-29.3547557522879,-66.8404642221305));
#23502=CARTESIAN_POINT('Ctrl Pts',(46.6715728752538,-29.8939769234005,-66.5984244836407));
#23503=CARTESIAN_POINT('',(40.5,-73.,0.));
#23504=CARTESIAN_POINT('',(43.5,-73.,-8.93992163377568E-15));
#23505=CARTESIAN_POINT('Origin',(40.5,0.,0.));
#23506=CARTESIAN_POINT('Origin',(46.5,0.,-4.16333634234434E-16));
#23507=CARTESIAN_POINT('',(48.0857864376272,31.3127256445526,-65.2941922269197));
#23508=CARTESIAN_POINT('',(48.2311293298322,31.4232291358174,-64.9999999991507));
#23509=CARTESIAN_POINT('Ctrl Pts',(48.0857864376269,31.3127256445523,-65.29419222692));
#23510=CARTESIAN_POINT('Ctrl Pts',(48.1379693066647,31.3533479964789,-65.1994073067213));
#23511=CARTESIAN_POINT('Ctrl Pts',(48.1867097226798,31.3902501843818,-65.1012175564133));
#23512=CARTESIAN_POINT('Ctrl Pts',(48.2311293298322,31.4232291358174,-64.9999999991507));
#23513=CARTESIAN_POINT('',(48.0857864376269,30.6065287460451,65.6281854386855));
#23514=CARTESIAN_POINT('Origin',(48.0857864376269,0.,-4.16333634234434E-16));
#23515=CARTESIAN_POINT('',(48.5,29.0466953015038,65.0006740405345));
#23516=CARTESIAN_POINT('Ctrl Pts',(48.5,29.0466953013294,65.0006740505758));
#23517=CARTESIAN_POINT('Ctrl Pts',(48.4999999991287,29.2503863229646,65.0042110518181));
#23518=CARTESIAN_POINT('Ctrl Pts',(48.4947069418067,29.4582861404335,65.022120804513));
#23519=CARTESIAN_POINT('Ctrl Pts',(48.4614290981404,29.8188223615094,65.093668653765));
#23520=CARTESIAN_POINT('Ctrl Pts',(48.4373072643951,29.9796369412407,65.1412137624121));
#23521=CARTESIAN_POINT('Ctrl Pts',(48.3647629082104,30.2376016389712,65.2605302175309));
#23522=CARTESIAN_POINT('Ctrl Pts',(48.3231006418053,30.3406889822552,65.3242242320176));
#23523=CARTESIAN_POINT('Ctrl Pts',(48.2166759088974,30.5047262139872,65.4694903771709));
#23524=CARTESIAN_POINT('Ctrl Pts',(48.1563934129581,30.5653976622582,65.5459946552306));
#23525=CARTESIAN_POINT('Ctrl Pts',(48.0857864376269,30.6065287460451,65.6281854386855));
#23526=CARTESIAN_POINT('',(48.5,31.2619954337637,-63.9647228889383));
#23527=CARTESIAN_POINT('Origin',(48.5,0.,-4.16333634234434E-16));
#23528=CARTESIAN_POINT('Ctrl Pts',(48.2311293298322,31.4232291358174,-64.9999999991507));
#23529=CARTESIAN_POINT('Ctrl Pts',(48.2715171949672,31.4532147553691,-64.9079694452346));
#23530=CARTESIAN_POINT('Ctrl Pts',(48.3105502826012,31.4736788152368,-64.8122557494851));
#23531=CARTESIAN_POINT('Ctrl Pts',(48.3948971358411,31.4925877457303,-64.5781032722722));
#23532=CARTESIAN_POINT('Ctrl Pts',(48.4357433706305,31.479360669589,-64.4404239144226));
#23533=CARTESIAN_POINT('Ctrl Pts',(48.4876874516577,31.3991541018519,-64.1828530709004));
#23534=CARTESIAN_POINT('Ctrl Pts',(48.5,31.3397623793345,-64.0691058819803));
#23535=CARTESIAN_POINT('Ctrl Pts',(48.5,31.261995430077,-63.9647228854568));
#23536=CARTESIAN_POINT('Origin',(48.5,53.,0.));
#23537=CARTESIAN_POINT('',(48.5,28.9686269665969,65.));
#23538=CARTESIAN_POINT('Ctrl Pts',(48.5,29.0466953013294,65.0006740505758));
#23539=CARTESIAN_POINT('Ctrl Pts',(48.5,29.0203628803793,65.0002168001558));
#23540=CARTESIAN_POINT('Ctrl Pts',(48.5,28.9943212164188,65.));
#23541=CARTESIAN_POINT('Ctrl Pts',(48.5,28.9686269665969,65.));
#23542=CARTESIAN_POINT('',(48.5,20.6143782776615,65.));
#23543=CARTESIAN_POINT('',(48.5,26.5,65.));
#23544=CARTESIAN_POINT('',(48.5,20.6143782776615,-77.));
#23545=CARTESIAN_POINT('',(48.5,20.6143782776615,-63.));
#23546=CARTESIAN_POINT('',(48.5,20.6143782776615,-77.));
#23547=CARTESIAN_POINT('',(48.5,28.9686269665969,-63.));
#23548=CARTESIAN_POINT('',(48.5,26.5,-63.));
#23549=CARTESIAN_POINT('Ctrl Pts',(48.5,28.9686269665969,-63.));
#23550=CARTESIAN_POINT('Ctrl Pts',(48.5,29.3555738612142,-63.));
#23551=CARTESIAN_POINT('Ctrl Pts',(48.5,29.8155012575532,-63.0638354527098));
#23552=CARTESIAN_POINT('Ctrl Pts',(48.5,30.4573223491148,-63.2950310532685));
#23553=CARTESIAN_POINT('Ctrl Pts',(48.5,30.7662183987536,-63.4685459818617));
#23554=CARTESIAN_POINT('Ctrl Pts',(48.5,31.0821687424774,-63.7502960288675));
#23555=CARTESIAN_POINT('Ctrl Pts',(48.5,31.1786502720937,-63.8528525155057));
#23556=CARTESIAN_POINT('Ctrl Pts',(48.5,31.2619954330609,-63.964722889462));
#23557=CARTESIAN_POINT('',(48.5,31.,-49.1935750346352));
#23558=CARTESIAN_POINT('Origin',(48.5,31.,-53.6935750346352));
#23559=CARTESIAN_POINT('',(48.5,31.,58.1935750346352));
#23560=CARTESIAN_POINT('Origin',(48.5,31.,53.6935750346352));
#23561=CARTESIAN_POINT('',(48.5,62.,4.5));
#23562=CARTESIAN_POINT('Origin',(48.5,62.,0.));
#23563=CARTESIAN_POINT('Origin',(46.6715728752538,0.,0.));
#23564=CARTESIAN_POINT('Ctrl Pts',(48.0857864376269,30.6065287460451,65.6281854386856));
#23565=CARTESIAN_POINT('Ctrl Pts',(47.9999019239268,30.6339819569562,65.7101473578198));
#23566=CARTESIAN_POINT('Ctrl Pts',(47.9086549996909,30.6381886023579,65.791498635381));
#23567=CARTESIAN_POINT('Ctrl Pts',(47.6860457696345,30.606362608182,65.9774777549062));
#23568=CARTESIAN_POINT('Ctrl Pts',(47.5541390304854,30.5542981832038,66.0778114080422));
#23569=CARTESIAN_POINT('Ctrl Pts',(47.244379598631,30.3822100790379,66.2963162354507));
#23570=CARTESIAN_POINT('Ctrl Pts',(47.0481190367442,30.2289549206708,66.4196105770725));
#23571=CARTESIAN_POINT('Ctrl Pts',(46.7881288893781,29.9653860177436,66.5635667604956));
#23572=CARTESIAN_POINT('Ctrl Pts',(46.7298294631265,29.9024655481068,66.5946537999311));
#23573=CARTESIAN_POINT('Ctrl Pts',(46.6715728753514,29.8356437962676,66.6245777417181));
#23574=CARTESIAN_POINT('Ctrl Pts',(46.6715728752538,29.8939769234005,-66.5984244836407));
#23575=CARTESIAN_POINT('Ctrl Pts',(46.9438337493957,30.2460388819865,-66.440394738235));
#23576=CARTESIAN_POINT('Ctrl Pts',(47.2187895890396,30.5412296642388,-66.2435626590178));
#23577=CARTESIAN_POINT('Ctrl Pts',(47.7030292472569,31.0032903130161,-65.7928556068471));
#23578=CARTESIAN_POINT('Ctrl Pts',(47.9098828723248,31.1757914999452,-65.5549458876211));
#23579=CARTESIAN_POINT('Ctrl Pts',(48.0857864376305,31.3127256445551,-65.2941922269146));
#23580=CARTESIAN_POINT('Origin',(40.5,0.,0.));
#23581=CARTESIAN_POINT('',(38.5,-71.,-1.73899845478924E-14));
#23582=CARTESIAN_POINT('Origin',(40.5,-71.,0.));
#23583=CARTESIAN_POINT('Origin',(38.5,0.,0.));
#23584=CARTESIAN_POINT('Origin',(38.5,72.,0.));
#23585=CARTESIAN_POINT('',(38.5,-31.,-49.1935750346352));
#23586=CARTESIAN_POINT('Origin',(38.5,-31.,-53.6935750346352));
#23587=CARTESIAN_POINT('',(38.5,62.,4.5));
#23588=CARTESIAN_POINT('Origin',(38.5,62.,0.));
#23589=CARTESIAN_POINT('',(38.5,31.,58.1935750346352));
#23590=CARTESIAN_POINT('Origin',(38.5,31.,53.6935750346352));
#23591=CARTESIAN_POINT('',(38.5,-31.,58.1935750346352));
#23592=CARTESIAN_POINT('Origin',(38.5,-31.,53.6935750346352));
#23593=CARTESIAN_POINT('',(38.5,-62.,4.50000000000001));
#23594=CARTESIAN_POINT('Origin',(38.5,-62.,7.59281015471359E-15));
#23595=CARTESIAN_POINT('',(38.5,31.,-49.1935750346352));
#23596=CARTESIAN_POINT('Origin',(38.5,31.,-53.6935750346352));
#23597=CARTESIAN_POINT('',(38.5,-6.2659657814934E-15,51.1654934782503));
#23598=CARTESIAN_POINT('Origin',(38.5,0.,0.));
#23599=CARTESIAN_POINT('Origin',(53.,-25.,67.));
#23600=CARTESIAN_POINT('',(53.,-31.,65.));
#23601=CARTESIAN_POINT('Origin',(53.,-25.,65.));
#23602=CARTESIAN_POINT('',(53.,-33.,67.));
#23603=CARTESIAN_POINT('Origin',(53.,-31.,67.));
#23604=CARTESIAN_POINT('Origin',(53.,-25.,67.));
#23605=CARTESIAN_POINT('Origin',(57.,-31.,67.));
#23606=CARTESIAN_POINT('',(69.,-31.,65.));
#23607=CARTESIAN_POINT('',(69.,-33.,67.));
#23608=CARTESIAN_POINT('Origin',(69.,-31.,67.));
#23609=CARTESIAN_POINT('',(57.,-33.,67.));
#23610=CARTESIAN_POINT('',(57.,-31.,65.));
#23611=CARTESIAN_POINT('Origin',(69.,-25.,67.));
#23612=CARTESIAN_POINT('',(75.,-25.,65.));
#23613=CARTESIAN_POINT('',(77.,-25.,67.));
#23614=CARTESIAN_POINT('Origin',(75.,-25.,67.));
#23615=CARTESIAN_POINT('Origin',(69.,-25.,67.));
#23616=CARTESIAN_POINT('Origin',(69.,-25.,65.));
#23617=CARTESIAN_POINT('Origin',(75.,-7.,67.));
#23618=CARTESIAN_POINT('',(75.,-19.2915026221292,65.));
#23619=CARTESIAN_POINT('',(77.,-14.,67.));
#23620=CARTESIAN_POINT('Ctrl Pts',(77.,-14.,67.));
#23621=CARTESIAN_POINT('Ctrl Pts',(77.,-14.8922724470027,66.5538637764986));
#23622=CARTESIAN_POINT('Ctrl Pts',(76.8431824332822,-15.8525818385793,66.0701256324549));
#23623=CARTESIAN_POINT('Ctrl Pts',(76.1700160324087,-17.6794947918718,65.2991643782353));
#23624=CARTESIAN_POINT('Ctrl Pts',(75.6598443730912,-18.5433094298986,65.));
#23625=CARTESIAN_POINT('Ctrl Pts',(75.,-19.2915026221292,65.));
#23626=CARTESIAN_POINT('',(77.,-7.,67.));
#23627=CARTESIAN_POINT('',(75.,-7.,65.));
#23628=CARTESIAN_POINT('Origin',(77.,-14.,-77.));
#23629=CARTESIAN_POINT('',(77.,-14.,-77.));
#23630=CARTESIAN_POINT('',(77.,14.,67.));
#23631=CARTESIAN_POINT('',(77.,14.,-77.));
#23632=CARTESIAN_POINT('',(77.,25.,67.));
#23633=CARTESIAN_POINT('',(77.,-7.,67.));
#23634=CARTESIAN_POINT('',(77.,25.,80.));
#23635=CARTESIAN_POINT('',(77.,25.,65.));
#23636=CARTESIAN_POINT('',(77.,-25.,80.));
#23637=CARTESIAN_POINT('',(77.,-7.,80.));
#23638=CARTESIAN_POINT('',(77.,-25.,65.));
#23639=CARTESIAN_POINT('Origin',(61.,0.,65.));
#23640=CARTESIAN_POINT('',(53.,-22.,65.));
#23641=CARTESIAN_POINT('Origin',(53.,-14.,65.));
#23642=CARTESIAN_POINT('',(69.,-22.,65.));
#23643=CARTESIAN_POINT('',(57.,-22.,65.));
#23644=CARTESIAN_POINT('Origin',(69.,-14.,65.));
#23645=CARTESIAN_POINT('Origin',(75.,-7.,80.));
#23646=CARTESIAN_POINT('Origin',(75.,-25.,80.));
#23647=CARTESIAN_POINT('Origin',(75.,25.,80.));
#23648=CARTESIAN_POINT('Origin',(69.,25.,80.));
#23649=CARTESIAN_POINT('',(69.,33.,80.));
#23650=CARTESIAN_POINT('Origin',(69.,31.,80.));
#23651=CARTESIAN_POINT('Origin',(69.,25.,80.));
#23652=CARTESIAN_POINT('Origin',(65.,31.,80.));
#23653=CARTESIAN_POINT('',(53.,33.,80.));
#23654=CARTESIAN_POINT('Origin',(53.,31.,80.));
#23655=CARTESIAN_POINT('',(65.,33.,80.));
#23656=CARTESIAN_POINT('Origin',(53.,25.,80.));
#23657=CARTESIAN_POINT('',(45.,25.,80.));
#23658=CARTESIAN_POINT('Origin',(47.,25.,80.));
#23659=CARTESIAN_POINT('Origin',(53.,25.,80.));
#23660=CARTESIAN_POINT('Origin',(47.,7.,80.));
#23661=CARTESIAN_POINT('',(45.,-25.,80.));
#23662=CARTESIAN_POINT('Origin',(47.,-25.,80.));
#23663=CARTESIAN_POINT('',(45.,7.,80.));
#23664=CARTESIAN_POINT('Origin',(53.,-25.,80.));
#23665=CARTESIAN_POINT('',(53.,-33.,80.));
#23666=CARTESIAN_POINT('Origin',(53.,-31.,80.));
#23667=CARTESIAN_POINT('Origin',(53.,-25.,80.));
#23668=CARTESIAN_POINT('Origin',(57.,-31.,80.));
#23669=CARTESIAN_POINT('',(69.,-33.,80.));
#23670=CARTESIAN_POINT('Origin',(69.,-31.,80.));
#23671=CARTESIAN_POINT('',(57.,-33.,80.));
#23672=CARTESIAN_POINT('Origin',(69.,-25.,80.));
#23673=CARTESIAN_POINT('Origin',(69.,-25.,80.));
#23674=CARTESIAN_POINT('Origin',(53.,25.,65.));
#23675=CARTESIAN_POINT('',(53.,33.,67.));
#23676=CARTESIAN_POINT('',(53.,33.,65.));
#23677=CARTESIAN_POINT('Origin',(53.,25.,67.));
#23678=CARTESIAN_POINT('',(45.,25.,65.));
#23679=CARTESIAN_POINT('Origin',(69.,33.,65.));
#23680=CARTESIAN_POINT('',(69.,33.,67.));
#23681=CARTESIAN_POINT('',(69.,33.,65.));
#23682=CARTESIAN_POINT('',(65.,33.,67.));
#23683=CARTESIAN_POINT('Origin',(69.,25.,65.));
#23684=CARTESIAN_POINT('Origin',(69.,25.,67.));
#23685=CARTESIAN_POINT('Origin',(75.,-7.,67.));
#23686=CARTESIAN_POINT('',(75.,25.,65.));
#23687=CARTESIAN_POINT('Origin',(75.,25.,67.));
#23688=CARTESIAN_POINT('',(75.,19.2915026221292,65.));
#23689=CARTESIAN_POINT('Ctrl Pts',(75.,19.2915026221292,65.));
#23690=CARTESIAN_POINT('Ctrl Pts',(75.6598443730912,18.5433094298986,65.));
#23691=CARTESIAN_POINT('Ctrl Pts',(76.1700160324087,17.6794947918718,65.2991643782352));
#23692=CARTESIAN_POINT('Ctrl Pts',(76.8431824332822,15.8525818385793,66.0701256324549));
#23693=CARTESIAN_POINT('Ctrl Pts',(77.,14.8922724470027,66.5538637764986));
#23694=CARTESIAN_POINT('Ctrl Pts',(77.,14.,67.));
#23695=CARTESIAN_POINT('',(75.,-7.,65.));
#23696=CARTESIAN_POINT('Origin',(65.,31.,67.));
#23697=CARTESIAN_POINT('',(69.,31.,65.));
#23698=CARTESIAN_POINT('Origin',(69.,31.,67.));
#23699=CARTESIAN_POINT('',(53.,31.,65.));
#23700=CARTESIAN_POINT('',(65.,31.,65.));
#23701=CARTESIAN_POINT('Origin',(53.,31.,67.));
#23702=CARTESIAN_POINT('Origin',(53.,25.,67.));
#23703=CARTESIAN_POINT('Origin',(53.,25.,65.));
#23704=CARTESIAN_POINT('Origin',(69.,25.,67.));
#23705=CARTESIAN_POINT('Origin',(69.,25.,65.));
#23706=CARTESIAN_POINT('Origin',(61.,0.,65.));
#23707=CARTESIAN_POINT('',(69.,22.,65.));
#23708=CARTESIAN_POINT('Origin',(69.,14.,65.));
#23709=CARTESIAN_POINT('',(53.,22.,65.));
#23710=CARTESIAN_POINT('',(65.,22.,65.));
#23711=CARTESIAN_POINT('Origin',(53.,14.,65.));
#23712=CARTESIAN_POINT('Origin',(40.5,0.,0.));
#23713=CARTESIAN_POINT('',(39.5811541622525,-6.04841520276597E-15,49.3890581919384));
#23714=CARTESIAN_POINT('Origin',(40.5,-6.2659657814934E-15,51.1654934782503));
#23715=CARTESIAN_POINT('',(39.5811541622525,-49.3890581919384,-1.20968304055319E-14));
#23716=CARTESIAN_POINT('Origin',(39.5811541622525,0.,-3.02420760138299E-15));
#23717=CARTESIAN_POINT('Origin',(39.5811541622525,0.,-3.02420760138299E-15));
#23718=CARTESIAN_POINT('Origin',(44.2,0.,0.));
#23719=CARTESIAN_POINT('',(50.,-44.,-5.38844591624836E-15));
#23720=CARTESIAN_POINT('',(44.2,-47.,-5.75583995599256E-15));
#23721=CARTESIAN_POINT('Origin',(50.,0.,0.));
#23722=CARTESIAN_POINT('Ctrl Pts',(63.3333333333333,-6.59966329107444,-31.7128621774316));
#23723=CARTESIAN_POINT('Ctrl Pts',(62.1773896945574,-7.00835108389839,-33.1107619749047));
#23724=CARTESIAN_POINT('Ctrl Pts',(59.8510477373174,-7.17140712600759,-36.1605129538655));
#23725=CARTESIAN_POINT('Ctrl Pts',(57.183782288428,-6.08047773499016,-40.0089544705698));
#23726=CARTESIAN_POINT('Ctrl Pts',(55.3668393528774,-4.31463467556344,-42.7323184706779));
#23727=CARTESIAN_POINT('Ctrl Pts',(54.4252091326635,-2.64874627344738,-44.1725365377487));
#23728=CARTESIAN_POINT('Ctrl Pts',(53.9842199476096,-0.833885651421998,
-44.8528004529788));
#23729=CARTESIAN_POINT('Ctrl Pts',(53.9856754786376,0.833929869935245,-44.8504853272497));
#23730=CARTESIAN_POINT('Ctrl Pts',(54.3607684393205,2.38775013614543,-44.2719711995386));
#23731=CARTESIAN_POINT('Ctrl Pts',(55.2216130985053,4.14017606552555,-42.9536995244691));
#23732=CARTESIAN_POINT('Ctrl Pts',(57.007705320374,6.00979472992292,-40.2625095891802));
#23733=CARTESIAN_POINT('Ctrl Pts',(59.8499534347117,7.17041001211291,-36.1623598714334));
#23734=CARTESIAN_POINT('Ctrl Pts',(62.177413277237,7.00834274616208,-33.1107334560203));
#23735=CARTESIAN_POINT('Ctrl Pts',(63.3333333333333,6.59966329107444,-31.7128621774316));
#23736=CARTESIAN_POINT('Ctrl Pts',(63.1962492273341,-6.64812984154691,-31.5488996087769));
#23737=CARTESIAN_POINT('Ctrl Pts',(62.0093421297043,-7.04072991080625,-32.9391773083993));
#23738=CARTESIAN_POINT('Ctrl Pts',(59.6306065410736,-7.14633030805639,-35.9670953227804));
#23739=CARTESIAN_POINT('Ctrl Pts',(56.9648786541832,-5.94451145070926,-39.762309829984));
#23740=CARTESIAN_POINT('Ctrl Pts',(55.2199817816534,-4.11869812402828,-42.409002614623));
#23741=CARTESIAN_POINT('Ctrl Pts',(54.3627838804906,-2.46985625068407,-43.7767782773241));
#23742=CARTESIAN_POINT('Ctrl Pts',(53.9869023625283,-0.76523709649401,-44.4022656717365));
#23743=CARTESIAN_POINT('Ctrl Pts',(53.9876569730852,0.765132497213866,-44.4005227560803));
#23744=CARTESIAN_POINT('Ctrl Pts',(54.308269419325,2.22454580031585,-43.8679449989279));
#23745=CARTESIAN_POINT('Ctrl Pts',(55.0839094544005,3.93929433219883,-42.6222903885058));
#23746=CARTESIAN_POINT('Ctrl Pts',(56.7877816472993,5.86696731444184,-40.0130840027767));
#23747=CARTESIAN_POINT('Ctrl Pts',(59.6300671008111,7.14497282840818,-35.9685572168257));
#23748=CARTESIAN_POINT('Ctrl Pts',(62.0093663440767,7.04072190127938,-32.9391489450152));
#23749=CARTESIAN_POINT('Ctrl Pts',(63.1962492273341,6.64812984154691,-31.5488996087769));
#23750=CARTESIAN_POINT('Ctrl Pts',(62.9463311105498,-6.81360008562125,-31.2209941996293));
#23751=CARTESIAN_POINT('Ctrl Pts',(61.6902590726639,-7.19193133539315,-32.5959957954705));
#23752=CARTESIAN_POINT('Ctrl Pts',(59.1806872784941,-7.22378666187567,-35.5805956265476));
#23753=CARTESIAN_POINT('Ctrl Pts',(56.4330578953553,-5.84073365634425,-39.2697533297976));
#23754=CARTESIAN_POINT('Ctrl Pts',(54.7292640216373,-3.8844953708936,-41.7632573520683));
#23755=CARTESIAN_POINT('Ctrl Pts',(53.965245234288,-2.22567623138461,-42.9858057638349));
#23756=CARTESIAN_POINT('Ctrl Pts',(53.6755658826225,-0.666505530006447,
-43.501384002397));
#23757=CARTESIAN_POINT('Ctrl Pts',(53.6752225587962,0.6661183946874,-43.5007858534596));
#23758=CARTESIAN_POINT('Ctrl Pts',(53.9239413145957,2.00085102106527,-43.0603333980273));
#23759=CARTESIAN_POINT('Ctrl Pts',(54.6011329384079,3.69297684653767,-41.9602076461288));
#23760=CARTESIAN_POINT('Ctrl Pts',(56.2489427064185,5.75229252847979,-39.5150983136102));
#23761=CARTESIAN_POINT('Ctrl Pts',(59.1809320219284,7.22165892747492,-35.5812660792604));
#23762=CARTESIAN_POINT('Ctrl Pts',(61.6902846980866,7.19192361696785,-32.5959677437378));
#23763=CARTESIAN_POINT('Ctrl Pts',(62.9463311105498,6.81360008562125,-31.2209941996293));
#23764=CARTESIAN_POINT('Ctrl Pts',(62.7061595886978,-7.20521258113835,-30.8184466564059));
#23765=CARTESIAN_POINT('Ctrl Pts',(61.3525918084501,-7.61031511383114,-32.1841418341022));
#23766=CARTESIAN_POINT('Ctrl Pts',(58.6397135353473,-7.65456619081017,-35.1410675266432));
#23767=CARTESIAN_POINT('Ctrl Pts',(55.637456029258,-6.19006620504293,-38.7682879574204));
#23768=CARTESIAN_POINT('Ctrl Pts',(53.7521005295524,-4.10520928504339,-41.1834647166237));
#23769=CARTESIAN_POINT('Ctrl Pts',(52.896526947302,-2.33958599845526,-42.3384335758014));
#23770=CARTESIAN_POINT('Ctrl Pts',(52.5690532918678,-0.69710377877861,-42.8061313896708));
#23771=CARTESIAN_POINT('Ctrl Pts',(52.5687476409763,0.696653785021548,-42.8059981646796));
#23772=CARTESIAN_POINT('Ctrl Pts',(52.8497229834458,2.1025880600763,-42.405744459455));
#23773=CARTESIAN_POINT('Ctrl Pts',(53.6092348807766,3.90049216650729,-41.3724241088537));
#23774=CARTESIAN_POINT('Ctrl Pts',(55.4364449073139,6.09674247261476,-39.0101551866323));
#23775=CARTESIAN_POINT('Ctrl Pts',(58.6398745251078,7.65211573990002,-35.1414067287986));
#23776=CARTESIAN_POINT('Ctrl Pts',(61.3526194229065,7.61030684923857,-32.1841139722319));
#23777=CARTESIAN_POINT('Ctrl Pts',(62.7061595886978,7.20521258113835,-30.8184466564059));
#23778=CARTESIAN_POINT('Ctrl Pts',(62.5904039193511,-7.6583127936691,-30.5250624561552));
#23779=CARTESIAN_POINT('Ctrl Pts',(61.1584933846712,-8.11585881641404,-31.8989848492516));
#23780=CARTESIAN_POINT('Ctrl Pts',(58.2791899818164,-8.24150163010199,-34.8759107492543));
#23781=CARTESIAN_POINT('Ctrl Pts',(55.0265173915859,-6.82101714568871,-38.556644545297));
#23782=CARTESIAN_POINT('Ctrl Pts',(52.8925220087755,-4.67295100884693,-41.0601803137195));
#23783=CARTESIAN_POINT('Ctrl Pts',(51.8521821945375,-2.76155870131978,-42.3047892112534));
#23784=CARTESIAN_POINT('Ctrl Pts',(51.4059828265007,-0.845790495339543,
-42.843015607466));
#23785=CARTESIAN_POINT('Ctrl Pts',(51.4066822856346,0.845549070264003,-42.8421168527233));
#23786=CARTESIAN_POINT('Ctrl Pts',(51.7875421911392,2.48554240511298,-42.382782492684));
#23787=CARTESIAN_POINT('Ctrl Pts',(52.7260106805419,4.46114907550238,-41.2588268883627));
#23788=CARTESIAN_POINT('Ctrl Pts',(54.8102735447582,6.7299823631145,-38.8010166853369));
#23789=CARTESIAN_POINT('Ctrl Pts',(58.2786008454734,8.23949994358309,-34.8767640575889));
#23790=CARTESIAN_POINT('Ctrl Pts',(61.1585225974167,8.11584948190943,-31.8989568195359));
#23791=CARTESIAN_POINT('Ctrl Pts',(62.5904039193511,7.6583127936691,-30.5250624561552));
#23792=CARTESIAN_POINT('Ctrl Pts',(62.5777174765495,-7.9634392868377,-30.3968807187894));
#23793=CARTESIAN_POINT('Ctrl Pts',(61.1076965731432,-8.46164972651616,-31.7860405531774));
#23794=CARTESIAN_POINT('Ctrl Pts',(58.1491913574022,-8.6588051165908,-34.8022816412753));
#23795=CARTESIAN_POINT('Ctrl Pts',(54.770406003722,-7.30098646822153,-38.5745581184182));
#23796=CARTESIAN_POINT('Ctrl Pts',(52.4937591618684,-5.13053317476476,-41.2071453587244));
#23797=CARTESIAN_POINT('Ctrl Pts',(51.3345717216213,-3.11536681555036,-42.5713405178562));
#23798=CARTESIAN_POINT('Ctrl Pts',(50.80489364747,-0.973086475418704,-43.1985149672608));
#23799=CARTESIAN_POINT('Ctrl Pts',(50.8063933838826,0.973031903179425,-43.1967026130617));
#23800=CARTESIAN_POINT('Ctrl Pts',(51.2573520876146,2.80710953729802,-42.6627697753439));
#23801=CARTESIAN_POINT('Ctrl Pts',(52.3130437902742,4.91587606463395,-41.419363544675));
#23802=CARTESIAN_POINT('Ctrl Pts',(54.5468818639601,7.21342605270668,-38.8237752884765));
#23803=CARTESIAN_POINT('Ctrl Pts',(58.1480381345749,8.65729203243944,-34.8037642919162));
#23804=CARTESIAN_POINT('Ctrl Pts',(61.1077265633873,8.46163956240716,-31.7860122125991));
#23805=CARTESIAN_POINT('Ctrl Pts',(62.5777174765495,7.9634392868377,-30.3968807187894));
#23806=CARTESIAN_POINT('Ctrl Pts',(62.5857864376269,-8.11974451941452,-30.3467059609741));
#23807=CARTESIAN_POINT('Ctrl Pts',(61.0995731877722,-8.63911281829804,-31.74623454857));
#23808=CARTESIAN_POINT('Ctrl Pts',(58.1085620998922,-8.87362866313132,-34.7889742482164));
#23809=CARTESIAN_POINT('Ctrl Pts',(54.6792208084628,-7.54849040484405,-38.6195517001502));
#23810=CARTESIAN_POINT('Ctrl Pts',(52.3431513198979,-5.36616124891415,-41.3291120736047));
#23811=CARTESIAN_POINT('Ctrl Pts',(51.1324838939085,-3.29727471161762,-42.7617756824825));
#23812=CARTESIAN_POINT('Ctrl Pts',(50.5654977988392,-1.03845908333126,-43.438457668019));
#23813=CARTESIAN_POINT('Ctrl Pts',(50.5673691958753,1.03851583598142,-43.4361543056794));
#23814=CARTESIAN_POINT('Ctrl Pts',(51.0496315738962,2.97241028941536,-42.8606883506125));
#23815=CARTESIAN_POINT('Ctrl Pts',(52.1564318499909,5.14998354500412,-41.5493290169032));
#23816=CARTESIAN_POINT('Ctrl Pts',(54.4528361352506,7.46272682506624,-38.871938946387));
#23817=CARTESIAN_POINT('Ctrl Pts',(58.1071551393991,8.87236958524201,-34.7908086217603));
#23818=CARTESIAN_POINT('Ctrl Pts',(61.0996035083602,8.63910222254254,-31.7462059964563));
#23819=CARTESIAN_POINT('Ctrl Pts',(62.5857864376269,8.11974451941452,-30.3467059609741));
#23820=CARTESIAN_POINT('',(62.0001023839998,8.30322829225476,-30.9040904042794));
#23821=CARTESIAN_POINT('',(62.0001200040293,-8.30324353871505,-30.9040671432868));
#23822=CARTESIAN_POINT('Ctrl Pts',(62.0001012510352,8.30322731523632,-30.9040918407253));
#23823=CARTESIAN_POINT('Ctrl Pts',(61.5941099144469,8.41601233957157,-31.294418998263));
#23824=CARTESIAN_POINT('Ctrl Pts',(61.1881353144704,8.49983265749143,-31.6926113194296));
#23825=CARTESIAN_POINT('Ctrl Pts',(60.7837478174969,8.55624046373246,-32.0961848387561));
#23826=CARTESIAN_POINT('Ctrl Pts',(60.3590806981778,8.61547706417824,-32.5199971602756));
#23827=CARTESIAN_POINT('Ctrl Pts',(59.9361642491327,8.64448288128927,-32.9497439708323));
#23828=CARTESIAN_POINT('Ctrl Pts',(59.5168590726499,8.64506377982343,-33.3825098937528));
#23829=CARTESIAN_POINT('Ctrl Pts',(59.2963181027409,8.6453693136764,-33.6101307812053));
#23830=CARTESIAN_POINT('Ctrl Pts',(59.0767768036617,8.63781144485083,-33.8385862524986));
#23831=CARTESIAN_POINT('Ctrl Pts',(58.858509746758,8.62265371547609,-34.0674479590845));
#23832=CARTESIAN_POINT('Ctrl Pts',(58.6277262935084,8.60662677500166,-34.3094336059876));
#23833=CARTESIAN_POINT('Ctrl Pts',(58.39818772758,8.58201871678512,-34.5520800845962));
#23834=CARTESIAN_POINT('Ctrl Pts',(58.1701981943553,8.5491694637154,-34.7948922255947));
#23835=CARTESIAN_POINT('Ctrl Pts',(57.8329926670629,8.50058412058207,-35.1540209754116));
#23836=CARTESIAN_POINT('Ctrl Pts',(57.4991770870744,8.43396948207508,-35.5135109022731));
#23837=CARTESIAN_POINT('Ctrl Pts',(57.1696794849973,8.34871184595084,-35.8717709918078));
#23838=CARTESIAN_POINT('Ctrl Pts',(56.8493772762383,8.26583352151987,-36.2200330042316));
#23839=CARTESIAN_POINT('Ctrl Pts',(56.5331556928524,8.16533894646567,-36.5671321395276));
#23840=CARTESIAN_POINT('Ctrl Pts',(56.2218388148571,8.04669241324987,-36.9116334654208));
#23841=CARTESIAN_POINT('Ctrl Pts',(55.9343240716864,7.93711715428765,-37.2297954965771));
#23842=CARTESIAN_POINT('Ctrl Pts',(55.6509928326656,7.81206045781843,-37.5457413038118));
#23843=CARTESIAN_POINT('Ctrl Pts',(55.3724670951342,7.67111227501838,-37.858371532471));
#23844=CARTESIAN_POINT('Ctrl Pts',(55.1989249042423,7.58329110394045,-38.0531633506399));
#23845=CARTESIAN_POINT('Ctrl Pts',(55.0272477780776,7.48930072219156,-38.2466686113815));
#23846=CARTESIAN_POINT('Ctrl Pts',(54.8575797184335,7.38904192488208,-38.4386296303125));
#23847=CARTESIAN_POINT('Ctrl Pts',(54.6442441141775,7.26297947593995,-38.679995742786));
#23848=CARTESIAN_POINT('Ctrl Pts',(54.4345041567674,7.12692432952911,-38.9185103314235));
#23849=CARTESIAN_POINT('Ctrl Pts',(54.2285146699767,6.98061592018927,-39.1538065157717));
#23850=CARTESIAN_POINT('Ctrl Pts',(54.1954395384656,6.9571236053363,-39.1915873382915));
#23851=CARTESIAN_POINT('Ctrl Pts',(54.1624611267774,6.93336683779831,-39.2292851714087));
#23852=CARTESIAN_POINT('Ctrl Pts',(54.1295801071056,6.90934441644494,-39.2668984787726));
#23853=CARTESIAN_POINT('Ctrl Pts',(53.9349114980075,6.76712220440003,-39.4895840980498));
#23854=CARTESIAN_POINT('Ctrl Pts',(53.7436555827443,6.61559218141993,-39.7093077515375));
#23855=CARTESIAN_POINT('Ctrl Pts',(53.5567634172599,6.45410520199659,-39.9248076943406));
#23856=CARTESIAN_POINT('Ctrl Pts',(53.3801976129847,6.30154086989652,-40.1284006091302));
#23857=CARTESIAN_POINT('Ctrl Pts',(53.2075261217369,6.1400895378134,-40.3282244049943));
#23858=CARTESIAN_POINT('Ctrl Pts',(53.0395671024636,5.96916334439465,-40.5231997797519));
#23859=CARTESIAN_POINT('Ctrl Pts',(52.8822480606121,5.80906509487933,-40.7058237273925));
#23860=CARTESIAN_POINT('Ctrl Pts',(52.7290630593257,5.64065439307646,-40.8841944917208));
#23861=CARTESIAN_POINT('Ctrl Pts',(52.580704568405,5.46341141043919,-41.0574035177952));
#23862=CARTESIAN_POINT('Ctrl Pts',(52.5706706209874,5.45142391476649,-41.0691181844051));
#23863=CARTESIAN_POINT('Ctrl Pts',(52.5606587602156,5.43939600328583,-41.0808092299468));
#23864=CARTESIAN_POINT('Ctrl Pts',(52.5506692043932,5.42732750858862,-41.0924763687869));
#23865=CARTESIAN_POINT('Ctrl Pts',(52.326146367373,5.15607894497275,-41.3547041553726));
#23866=CARTESIAN_POINT('Ctrl Pts',(52.1134246130853,4.86497441262733,-41.604231853927));
#23867=CARTESIAN_POINT('Ctrl Pts',(51.9150764404737,4.55261153092244,-41.8377049019999));
#23868=CARTESIAN_POINT('Ctrl Pts',(51.6817907972624,4.18522838433518,-42.1123023912283));
#23869=CARTESIAN_POINT('Ctrl Pts',(51.4683897034793,3.78844091406138,-42.3646895021457));
#23870=CARTESIAN_POINT('Ctrl Pts',(51.2842097158458,3.36345268041168,-42.5830775379464));
#23871=CARTESIAN_POINT('Ctrl Pts',(51.2218736018392,3.21961449622777,-42.6569914396263));
#23872=CARTESIAN_POINT('Ctrl Pts',(51.1628846200672,3.07254551732303,-42.7270109645469));
#23873=CARTESIAN_POINT('Ctrl Pts',(51.1076045454045,2.92229120412496,-42.79267942641));
#23874=CARTESIAN_POINT('Ctrl Pts',(51.0777650817789,2.84118588470146,-42.8281264060148));
#23875=CARTESIAN_POINT('Ctrl Pts',(51.0490066311153,2.7591539419897,-42.8623052012408));
#23876=CARTESIAN_POINT('Ctrl Pts',(51.0213793428822,2.67624432063873,-42.8951530087209));
#23877=CARTESIAN_POINT('Ctrl Pts',(50.93401383815,2.41406003185287,-42.9990273106656));
#23878=CARTESIAN_POINT('Ctrl Pts',(50.8579717898991,2.14313439968825,-43.0895777141708));
#23879=CARTESIAN_POINT('Ctrl Pts',(50.7950448077893,1.86551417994214,-43.1645736822976));
#23880=CARTESIAN_POINT('Ctrl Pts',(50.7635813167345,1.72670407006909,-43.202071666361));
#23881=CARTESIAN_POINT('Ctrl Pts',(50.7353969825947,1.58622028876809,-43.2356805725728));
#23882=CARTESIAN_POINT('Ctrl Pts',(50.7107183655813,1.44431884754542,-43.2651184376449));
#23883=CARTESIAN_POINT('Ctrl Pts',(50.6978982060417,1.37060324531452,-43.2804109528828));
#23884=CARTESIAN_POINT('Ctrl Pts',(50.6860241446869,1.29650507187844,-43.2945778164074));
#23885=CARTESIAN_POINT('Ctrl Pts',(50.6751281526797,1.22206025810523,-43.3075792459665));
#23886=CARTESIAN_POINT('Ctrl Pts',(50.6688327119529,1.1790478447136,-43.3150911576032));
#23887=CARTESIAN_POINT('Ctrl Pts',(50.6628638943807,1.13592001508024,-43.3222138760624));
#23888=CARTESIAN_POINT('Ctrl Pts',(50.657229426006,1.09269727206875,-43.3289378665353));
#23889=CARTESIAN_POINT('Ctrl Pts',(50.6538434412765,1.06672294085045,-43.332978590087));
#23890=CARTESIAN_POINT('Ctrl Pts',(50.6505780086374,1.04071306381805,-43.3368755494295));
#23891=CARTESIAN_POINT('Ctrl Pts',(50.6474343593728,1.01466909166829,-43.3406272068915));
#23892=CARTESIAN_POINT('Ctrl Pts',(50.6186694791588,0.776362691650125,-43.3749554567736));
#23893=CARTESIAN_POINT('Ctrl Pts',(50.600098342512,0.535203459559028,-43.3971213719785));
#23894=CARTESIAN_POINT('Ctrl Pts',(50.5917367840456,0.293243554386321,-43.4071042335405));
#23895=CARTESIAN_POINT('Ctrl Pts',(50.5883618175051,0.195581547070637,-43.4111336048456));
#23896=CARTESIAN_POINT('Ctrl Pts',(50.5866505170883,0.0977888671166625,
-43.4131777294003));
#23897=CARTESIAN_POINT('Ctrl Pts',(50.5866053901866,-2.17691642161351E-7,
-43.4132334956971));
#23898=CARTESIAN_POINT('Ctrl Pts',(50.586485167316,-0.260520750748842,-43.413382063049));
#23899=CARTESIAN_POINT('Ctrl Pts',(50.5982467100744,-0.521104937388154,
-43.3993625324755));
#23900=CARTESIAN_POINT('Ctrl Pts',(50.6219681403998,-0.77917008619531,-43.3710763758922));
#23901=CARTESIAN_POINT('Ctrl Pts',(50.6292153817941,-0.858012736203985,
-43.3624345443474));
#23902=CARTESIAN_POINT('Ctrl Pts',(50.6375791839474,-0.936620275249521,
-43.3524608025752));
#23903=CARTESIAN_POINT('Ctrl Pts',(50.6470624139535,-1.01491901366598,-43.3411515885966));
#23904=CARTESIAN_POINT('Ctrl Pts',(50.6472813846526,-1.01672695563096,-43.3408904553657));
#23905=CARTESIAN_POINT('Ctrl Pts',(50.6475009522024,-1.01853473295156,-43.3406286100948));
#23906=CARTESIAN_POINT('Ctrl Pts',(50.6477211161207,-1.02034234510595,-43.3403660533829));
#23907=CARTESIAN_POINT('Ctrl Pts',(50.673528927452,-1.23223225784476,-43.3095889208865));
#23908=CARTESIAN_POINT('Ctrl Pts',(50.7073631779969,-1.44168968568162,-43.2692082735287));
#23909=CARTESIAN_POINT('Ctrl Pts',(50.7484990707422,-1.64787039720256,-43.220143263679));
#23910=CARTESIAN_POINT('Ctrl Pts',(50.7921321138407,-1.86656728868811,-43.1680997671963));
#23911=CARTESIAN_POINT('Ctrl Pts',(50.84398110902,-2.08157734702968,-43.1062843533602));
#23912=CARTESIAN_POINT('Ctrl Pts',(50.9031825382286,-2.29183416733726,-43.0357934194958));
#23913=CARTESIAN_POINT('Ctrl Pts',(50.9292756216388,-2.3845050508477,-43.0047244767089));
#23914=CARTESIAN_POINT('Ctrl Pts',(50.9567969317084,-2.47625184720333,-42.9719703202599));
#23915=CARTESIAN_POINT('Ctrl Pts',(50.9856720258372,-2.56698024296232,-42.9376255742626));
#23916=CARTESIAN_POINT('Ctrl Pts',(51.0240408230126,-2.68753879073323,-42.8919887847397));
#23917=CARTESIAN_POINT('Ctrl Pts',(51.0648054205121,-2.8063940980028,-42.8435323454503));
#23918=CARTESIAN_POINT('Ctrl Pts',(51.1077731615943,-2.92331062745625,-42.7924952486978));
#23919=CARTESIAN_POINT('Ctrl Pts',(51.186049359457,-3.13630254098097,-42.6995187555632));
#23920=CARTESIAN_POINT('Ctrl Pts',(51.2716388252896,-3.34285777520948,-42.5979758659837));
#23921=CARTESIAN_POINT('Ctrl Pts',(51.3636626458657,-3.54285994422824,-42.4889780171507));
#23922=CARTESIAN_POINT('Ctrl Pts',(51.4604494463671,-3.75321384946142,-42.3743386446051));
#23923=CARTESIAN_POINT('Ctrl Pts',(51.5643534413362,-3.95631874229753,-42.2514532460909));
#23924=CARTESIAN_POINT('Ctrl Pts',(51.6743212746164,-4.15207844084002,-42.1216502585922));
#23925=CARTESIAN_POINT('Ctrl Pts',(51.793622211243,-4.36445250235611,-41.9808307341585));
#23926=CARTESIAN_POINT('Ctrl Pts',(51.9200593333631,-4.56818133269484,-41.8318704331003));
#23927=CARTESIAN_POINT('Ctrl Pts',(52.0522607572722,-4.76319042120215,-41.6764946462579));
#23928=CARTESIAN_POINT('Ctrl Pts',(52.1216221833531,-4.865504814479,-41.5949744490078));
#23929=CARTESIAN_POINT('Ctrl Pts',(52.1925699964374,-4.96541970222067,-41.5116886236485));
#23930=CARTESIAN_POINT('Ctrl Pts',(52.264904452046,-5.06292947504769,-41.4268878241172));
#23931=CARTESIAN_POINT('Ctrl Pts',(52.312104038938,-5.12655642788292,-41.3715537143584));
#23932=CARTESIAN_POINT('Ctrl Pts',(52.3599223500288,-5.18918440397153,-41.3155429681556));
#23933=CARTESIAN_POINT('Ctrl Pts',(52.4083099354638,-5.25081325409878,-41.25891856032));
#23934=CARTESIAN_POINT('Ctrl Pts',(52.7176297514124,-5.64477845006965,-40.8969444867553));
#23935=CARTESIAN_POINT('Ctrl Pts',(53.0502141797102,-5.99791651902043,-40.5098908689843));
#23936=CARTESIAN_POINT('Ctrl Pts',(53.3996025180074,-6.31470393262302,-40.1062255542024));
#23937=CARTESIAN_POINT('Ctrl Pts',(53.6358531256194,-6.52891033490946,-39.8332737540538));
#23938=CARTESIAN_POINT('Ctrl Pts',(53.8797866873093,-6.7264958123545,-39.5527271279448));
#23939=CARTESIAN_POINT('Ctrl Pts',(54.1293982844213,-6.90884160725303,-39.2672150609152));
#23940=CARTESIAN_POINT('Ctrl Pts',(54.2994416340632,-7.03306135551964,-39.0727151706752));
#23941=CARTESIAN_POINT('Ctrl Pts',(54.4721197328197,-7.15020875091379,-38.8759113199701));
#23942=CARTESIAN_POINT('Ctrl Pts',(54.6472513236306,-7.26040146543055,-38.6771162244914));
#23943=CARTESIAN_POINT('Ctrl Pts',(54.9699633495794,-7.46345172028084,-38.3107998579607));
#23944=CARTESIAN_POINT('Ctrl Pts',(55.3004435195228,-7.64300727204081,-37.9382715990561));
#23945=CARTESIAN_POINT('Ctrl Pts',(55.6375976843359,-7.79988175928238,-37.5614333033218));
#23946=CARTESIAN_POINT('Ctrl Pts',(56.0076859609607,-7.97208016193834,-37.1477844447593));
#23947=CARTESIAN_POINT('Ctrl Pts',(56.3858156688506,-8.1169486357207,-36.7289427228566));
#23948=CARTESIAN_POINT('Ctrl Pts',(56.7705126358147,-8.23551698557478,-36.3074625031452));
#23949=CARTESIAN_POINT('Ctrl Pts',(57.1943033398964,-8.36613450736868,-35.8431505526829));
#23950=CARTESIAN_POINT('Ctrl Pts',(57.6260640850358,-8.46483346777168,-35.3756366645352));
#23951=CARTESIAN_POINT('Ctrl Pts',(58.0637925846012,-8.53296150481107,-34.9083769250887));
#23952=CARTESIAN_POINT('Ctrl Pts',(58.0993721404169,-8.53849910471345,-34.8703970037525));
#23953=CARTESIAN_POINT('Ctrl Pts',(58.1349911067779,-8.54383472057116,-34.8324187822653));
#23954=CARTESIAN_POINT('Ctrl Pts',(58.1706483991881,-8.54896907247115,-34.7944441274998));
#23955=CARTESIAN_POINT('Ctrl Pts',(58.5551727492141,-8.60433736304228,-34.3849295947302));
#23956=CARTESIAN_POINT('Ctrl Pts',(58.944155818618,-8.63630043942602,-33.9758280479163));
#23957=CARTESIAN_POINT('Ctrl Pts',(59.3362796214209,-8.64327347910499,-33.5693510645206));
#23958=CARTESIAN_POINT('Ctrl Pts',(59.6583329109191,-8.64900047234121,-33.2355094342187));
#23959=CARTESIAN_POINT('Ctrl Pts',(59.9827515460476,-8.6381484172323,-32.9031110658833));
#23960=CARTESIAN_POINT('Ctrl Pts',(60.3086572343028,-8.60978376402087,-32.5735422953563));
#23961=CARTESIAN_POINT('Ctrl Pts',(60.6228690745861,-8.58243686519172,-32.255798808148));
#23962=CARTESIAN_POINT('Ctrl Pts',(60.938462675709,-8.53881140084064,-31.9406862056459));
#23963=CARTESIAN_POINT('Ctrl Pts',(61.254642507309,-8.47811729861641,-31.6294480076406));
#23964=CARTESIAN_POINT('Ctrl Pts',(61.5028961274628,-8.43046235958092,-31.3850743896462));
#23965=CARTESIAN_POINT('Ctrl Pts',(61.7515109191481,-8.37228568684251,-31.1430894138287));
#23966=CARTESIAN_POINT('Ctrl Pts',(62.0001008132074,-8.30322720641197,-30.9040914170777));
#23967=CARTESIAN_POINT('',(62.0088202634227,-8.3010477799695,-30.8955608315711));
#23968=CARTESIAN_POINT('Ctrl Pts',(62.0005099868911,-8.30357543269804,-30.9035738677768));
#23969=CARTESIAN_POINT('Ctrl Pts',(62.0033470639992,-8.30278347640663,-30.9008472871189));
#23970=CARTESIAN_POINT('Ctrl Pts',(62.0061841412741,-8.30199009465469,-30.8981210941654));
#23971=CARTESIAN_POINT('Ctrl Pts',(62.0090212182218,-8.30119528689782,-30.8953952897239));
#23972=CARTESIAN_POINT('',(63.3333333333333,-6.59966329107444,-31.7128621774316));
#23973=CARTESIAN_POINT('Ctrl Pts',(62.0085237301998,-8.30083011557419,-30.8958051086804));
#23974=CARTESIAN_POINT('Ctrl Pts',(62.0311590677664,-8.05644177174264,-30.9380272890384));
#23975=CARTESIAN_POINT('Ctrl Pts',(62.0981396788048,-7.82229842288598,-30.9982213762078));
#23976=CARTESIAN_POINT('Ctrl Pts',(62.315933348572,-7.37581872570051,-31.1536217805517));
#23977=CARTESIAN_POINT('Ctrl Pts',(62.4713648465707,-7.17154726294401,-31.249902943982));
#23978=CARTESIAN_POINT('Ctrl Pts',(62.8535438668198,-6.82510864454588,-31.4671224701204));
#23979=CARTESIAN_POINT('Ctrl Pts',(63.0820808101837,-6.68927586422443,-31.5880758676676));
#23980=CARTESIAN_POINT('Ctrl Pts',(63.3298258043247,-6.60090614371293,-31.7111212674739));
#23981=CARTESIAN_POINT('Ctrl Pts',(63.331579144709,-6.60028349041031,-31.7119917027094));
#23982=CARTESIAN_POINT('Ctrl Pts',(63.3333333333333,-6.59966329107444,-31.7128621774316));
#23983=CARTESIAN_POINT('',(54.0006369628663,-9.87019395503469E-7,-44.8274429326583));
#23984=CARTESIAN_POINT('Ctrl Pts',(63.3333333333333,-6.59966329107444,-31.7128621774316));
#23985=CARTESIAN_POINT('Ctrl Pts',(62.1773896945574,-7.00835108389839,-33.1107619749047));
#23986=CARTESIAN_POINT('Ctrl Pts',(59.8510477373174,-7.17140712600759,-36.1605129538655));
#23987=CARTESIAN_POINT('Ctrl Pts',(57.183782288428,-6.08047773499016,-40.0089544705698));
#23988=CARTESIAN_POINT('Ctrl Pts',(55.3668393528774,-4.31463467556344,-42.7323184706779));
#23989=CARTESIAN_POINT('Ctrl Pts',(54.4252091326635,-2.64874627344738,-44.1725365377487));
#23990=CARTESIAN_POINT('Ctrl Pts',(54.0472129322659,-1.09312894171435,-44.7556283321497));
#23991=CARTESIAN_POINT('Ctrl Pts',(54.0005126820376,-0.273223819838185,
-44.8276413098042));
#23992=CARTESIAN_POINT('Ctrl Pts',(54.0006369887046,5.63225172177384E-5,
-44.8274428914028));
#23993=CARTESIAN_POINT('',(63.3333333333333,6.59966329107444,-31.7128621774316));
#23994=CARTESIAN_POINT('Ctrl Pts',(54.0006369628663,-9.87019395576327E-7,
-44.8274429326583));
#23995=CARTESIAN_POINT('Ctrl Pts',(54.000759063025,0.273250808313191,-44.827247918389));
#23996=CARTESIAN_POINT('Ctrl Pts',(54.0481920300815,1.09290429704828,-44.7540646741929));
#23997=CARTESIAN_POINT('Ctrl Pts',(54.3607684393205,2.38775013614543,-44.2719711995386));
#23998=CARTESIAN_POINT('Ctrl Pts',(55.2216130985053,4.14017606552555,-42.9536995244691));
#23999=CARTESIAN_POINT('Ctrl Pts',(57.007705320374,6.00979472992292,-40.2625095891802));
#24000=CARTESIAN_POINT('Ctrl Pts',(59.8499534347117,7.17041001211291,-36.1623598714334));
#24001=CARTESIAN_POINT('Ctrl Pts',(62.177413277237,7.00834274616208,-33.1107334560203));
#24002=CARTESIAN_POINT('Ctrl Pts',(63.3333333333333,6.59966329107444,-31.7128621774316));
#24003=CARTESIAN_POINT('',(62.0088028665926,8.30103473250453,-30.8955848315571));
#24004=CARTESIAN_POINT('Ctrl Pts',(63.3333333333333,6.59966329107444,-31.7128621774316));
#24005=CARTESIAN_POINT('Ctrl Pts',(63.3315791446631,6.60028349042654,-31.7119917026866));
#24006=CARTESIAN_POINT('Ctrl Pts',(63.3298258160868,6.60090617043969,-31.7111212664723));
#24007=CARTESIAN_POINT('Ctrl Pts',(63.3280733522143,6.60153132813992,-31.7102508716682));
#24008=CARTESIAN_POINT('Ctrl Pts',(63.2635232041076,6.62455834899427,-31.6781908021871));
#24009=CARTESIAN_POINT('Ctrl Pts',(63.2001937780771,6.65092550213733,-31.6462071962042));
#24010=CARTESIAN_POINT('Ctrl Pts',(63.1383080680394,6.6804983322719,-31.6144426934177));
#24011=CARTESIAN_POINT('Ctrl Pts',(63.0761479782219,6.71020227808104,-31.58253735784));
#24012=CARTESIAN_POINT('Ctrl Pts',(63.015444088525,6.74314079497629,-31.5508526061538));
#24013=CARTESIAN_POINT('Ctrl Pts',(62.9564567516355,6.77921725541551,-31.5195350800571));
#24014=CARTESIAN_POINT('Ctrl Pts',(62.8977369868048,6.81513006966725,-31.4883596131781));
#24015=CARTESIAN_POINT('Ctrl Pts',(62.8407179621036,6.85415287127117,-31.4575476304171));
#24016=CARTESIAN_POINT('Ctrl Pts',(62.7856950660349,6.89622306178314,-31.4272524681983));
#24017=CARTESIAN_POINT('Ctrl Pts',(62.7691692946379,6.90885857173816,-31.4181535119268));
#24018=CARTESIAN_POINT('Ctrl Pts',(62.7528238671385,6.92176917986149,-31.4091012602555));
#24019=CARTESIAN_POINT('Ctrl Pts',(62.7366655328393,6.93495040659354,-31.4000991129422));
#24020=CARTESIAN_POINT('Ctrl Pts',(62.6833910901369,6.97840924927402,-31.3704188023133));
#24021=CARTESIAN_POINT('Ctrl Pts',(62.63226160359,7.02471404691096,-31.3413468098537));
#24022=CARTESIAN_POINT('Ctrl Pts',(62.5834883508633,7.07370394238452,-31.3130025833967));
#24023=CARTESIAN_POINT('Ctrl Pts',(62.5353508777631,7.12205523420339,-31.2850278357156));
#24024=CARTESIAN_POINT('Ctrl Pts',(62.4895084719016,7.17302268219252,-31.257761588209));
#24025=CARTESIAN_POINT('Ctrl Pts',(62.4462067271139,7.22647307749946,-31.2313344330245));
#24026=CARTESIAN_POINT('Ctrl Pts',(62.4102568378579,7.27084855939736,-31.2093941323071));
#24027=CARTESIAN_POINT('Ctrl Pts',(62.3760588170702,7.31693597573896,-31.1880323491785));
#24028=CARTESIAN_POINT('Ctrl Pts',(62.3437770329297,7.36466613151546,-31.1673352748822));
#24029=CARTESIAN_POINT('Ctrl Pts',(62.3208256261186,7.39860087990527,-31.1526202588253));
#24030=CARTESIAN_POINT('Ctrl Pts',(62.2988433325185,7.43336620520493,-31.1382414985304));
#24031=CARTESIAN_POINT('Ctrl Pts',(62.2778800856691,7.46892117258342,-31.1242222112547));
#24032=CARTESIAN_POINT('Ctrl Pts',(62.2423237652168,7.52922689825947,-31.1004437252946));
#24033=CARTESIAN_POINT('Ctrl Pts',(62.2098522421806,7.59153865793464,-31.077803087974));
#24034=CARTESIAN_POINT('Ctrl Pts',(62.180645578126,7.65563148244981,-31.0563991987818));
#24035=CARTESIAN_POINT('Ctrl Pts',(62.1580094653665,7.7053055020534,-31.0398104898372));
#24036=CARTESIAN_POINT('Ctrl Pts',(62.1373353088525,7.75604981429739,-31.0239650024763));
#24037=CARTESIAN_POINT('Ctrl Pts',(62.118725318096,7.80776250967515,-31.0089197705683));
#24038=CARTESIAN_POINT('Ctrl Pts',(62.0952037529992,7.87312329069713,-30.9899037803751));
#24039=CARTESIAN_POINT('Ctrl Pts',(62.0749785877622,7.94003185523155,-30.9721652566799));
#24040=CARTESIAN_POINT('Ctrl Pts',(62.0582301482953,8.00824501492773,-30.9557896333494));
#24041=CARTESIAN_POINT('Ctrl Pts',(62.0467738079755,8.0549044767425,-30.9445883083428));
#24042=CARTESIAN_POINT('Ctrl Pts',(62.0369450076869,8.10217425231307,-30.9340252251599));
#24043=CARTESIAN_POINT('Ctrl Pts',(62.0288121054035,8.14997249472371,-30.924136146721));
#24044=CARTESIAN_POINT('Ctrl Pts',(62.020307426509,8.19995572202247,-30.9137950121843));
#24045=CARTESIAN_POINT('Ctrl Pts',(62.013678947783,8.25038775318331,-30.9042177588782));
#24046=CARTESIAN_POINT('Ctrl Pts',(62.0089847266465,8.30116803958258,-30.8954413183826));
#24047=CARTESIAN_POINT('Ctrl Pts',(62.0089847242203,8.30116804026198,-30.8954413207137));
#24048=CARTESIAN_POINT('Ctrl Pts',(62.0061473048757,8.30196259736025,-30.8981675557624));
#24049=CARTESIAN_POINT('Ctrl Pts',(62.0033098833227,8.30275572690749,-30.900894181743));
#24050=CARTESIAN_POINT('Ctrl Pts',(62.0004724600677,8.30354742945956,-30.9036211978314));
#24051=CARTESIAN_POINT('Origin',(64.,-8.48528137423857,13.));
#24052=CARTESIAN_POINT('',(63.3333333333333,-6.59966329107444,31.7128621774316));
#24053=CARTESIAN_POINT('',(63.3333333333333,-6.59966329107444,13.));
#24054=CARTESIAN_POINT('',(62.,-8.48528137423857,-30.854497241083));
#24055=CARTESIAN_POINT('Ctrl Pts',(62.0085237301807,-8.30083011578128,-30.8958051086446));
#24056=CARTESIAN_POINT('Ctrl Pts',(62.0029032474376,-8.36151312820127,-30.885321101655));
#24057=CARTESIAN_POINT('Ctrl Pts',(62.,-8.42346268655744,-30.8714979705087));
#24058=CARTESIAN_POINT('Ctrl Pts',(62.,-8.48528137423856,-30.854497241083));
#24059=CARTESIAN_POINT('',(62.,-8.48528137423857,30.854497241083));
#24060=CARTESIAN_POINT('',(62.,-8.48528137423857,13.));
#24061=CARTESIAN_POINT('',(62.008849633308,-8.30100100727199,30.895526211557));
#24062=CARTESIAN_POINT('Ctrl Pts',(62.,-8.48528137423857,30.854497241083));
#24063=CARTESIAN_POINT('Ctrl Pts',(62.,-8.42347251099396,30.8714952686948));
#24064=CARTESIAN_POINT('Ctrl Pts',(62.0029020528202,-8.36152602610337,30.8853188733362));
#24065=CARTESIAN_POINT('Ctrl Pts',(62.0085237302078,-8.30083011548887,30.8958051086952));
#24066=CARTESIAN_POINT('Ctrl Pts',(63.3333333333333,-6.59966329107444,31.7128621774316));
#24067=CARTESIAN_POINT('Ctrl Pts',(63.3315791446588,-6.60028349042807,31.7119917026845));
#24068=CARTESIAN_POINT('Ctrl Pts',(63.3298258164317,-6.60090617028985,31.7111212659654));
#24069=CARTESIAN_POINT('Ctrl Pts',(63.3280733532319,-6.60153132770387,31.7102508701461));
#24070=CARTESIAN_POINT('Ctrl Pts',(63.2635050836892,-6.62456481132822,31.6781817505937));
#24071=CARTESIAN_POINT('Ctrl Pts',(63.2001586660833,-6.65094012635296,31.6461884495608));
#24072=CARTESIAN_POINT('Ctrl Pts',(63.1382571476502,-6.68052308701512,31.6144138631241));
#24073=CARTESIAN_POINT('Ctrl Pts',(63.0760620233079,-6.71024636300848,31.5824885662271));
#24074=CARTESIAN_POINT('Ctrl Pts',(63.0153251922965,-6.74320819450885,31.5507835985174));
#24075=CARTESIAN_POINT('Ctrl Pts',(62.956307457809,-6.77931199071329,31.5194460012486));
#24076=CARTESIAN_POINT('Ctrl Pts',(62.8976433010526,-6.81519948755522,31.4882961488439));
#24077=CARTESIAN_POINT('Ctrl Pts',(62.8406774425965,-6.85419187098811,31.4575088655831));
#24078=CARTESIAN_POINT('Ctrl Pts',(62.7857045379272,-6.89622665807325,31.4272371911452));
#24079=CARTESIAN_POINT('Ctrl Pts',(62.7691793523232,-6.90886256775612,31.4181373438361));
#24080=CARTESIAN_POINT('Ctrl Pts',(62.7528345382147,-6.92177360354981,31.4090841726496));
#24081=CARTESIAN_POINT('Ctrl Pts',(62.7366768459354,-6.93495528086646,31.4000810795403));
#24082=CARTESIAN_POINT('Ctrl Pts',(62.6833852217834,-6.97843135288908,31.3703868976057));
#24083=CARTESIAN_POINT('Ctrl Pts',(62.6322404130614,-7.02475569639747,31.3413011968834));
#24084=CARTESIAN_POINT('Ctrl Pts',(62.5834539692209,-7.07376700776111,31.3129436174977));
#24085=CARTESIAN_POINT('Ctrl Pts',(62.5353085615151,-7.12213432831251,31.2849586463951));
#24086=CARTESIAN_POINT('Ctrl Pts',(62.4894598137834,-7.17311907144123,31.2576823710423));
#24087=CARTESIAN_POINT('Ctrl Pts',(62.4461535426247,-7.22658757348273,31.231245525692));
#24088=CARTESIAN_POINT('Ctrl Pts',(62.4102361210531,-7.27093336168479,31.2093192943619));
#24089=CARTESIAN_POINT('Ctrl Pts',(62.3760682926572,-7.31698819323151,31.1879706493171));
#24090=CARTESIAN_POINT('Ctrl Pts',(62.3438140501227,-7.36468280083248,31.1672856002691));
#24091=CARTESIAN_POINT('Ctrl Pts',(62.3208649852281,-7.39861776748955,31.1525680779945));
#24092=CARTESIAN_POINT('Ctrl Pts',(62.2988851467792,-7.43338305818485,31.1381867524407));
#24093=CARTESIAN_POINT('Ctrl Pts',(62.2779244539186,-7.46893767670066,31.124164845081));
#24094=CARTESIAN_POINT('Ctrl Pts',(62.2423689479923,-7.52924877699471,31.1003795621449));
#24095=CARTESIAN_POINT('Ctrl Pts',(62.2098991175825,-7.5915653981267,31.0777322138085));
#24096=CARTESIAN_POINT('Ctrl Pts',(62.1806949586429,-7.65566232615891,31.0563217546863));
#24097=CARTESIAN_POINT('Ctrl Pts',(62.1580659155852,-7.70532827090699,31.0397317134404));
#24098=CARTESIAN_POINT('Ctrl Pts',(62.1373984273643,-7.75606357093779,31.0238846422908));
#24099=CARTESIAN_POINT('Ctrl Pts',(62.1187945868658,-7.80776633320906,31.0088375691922));
#24100=CARTESIAN_POINT('Ctrl Pts',(62.0952718368554,-7.87313945613236,30.9898120062223));
#24101=CARTESIAN_POINT('Ctrl Pts',(62.075047167823,-7.94006006372112,30.9720644712138));
#24102=CARTESIAN_POINT('Ctrl Pts',(62.0583009018868,-8.00828491614149,30.9556804706479));
#24103=CARTESIAN_POINT('Ctrl Pts',(62.0468531893068,-8.05492328342251,30.944480401922));
#24104=CARTESIAN_POINT('Ctrl Pts',(62.0370317732946,-8.10217104304868,30.9339180770259));
#24105=CARTESIAN_POINT('Ctrl Pts',(62.0289048874703,-8.1499465245071,30.9240292222972));
#24106=CARTESIAN_POINT('Ctrl Pts',(62.0204033521119,-8.19992445623345,30.9136844912469));
#24107=CARTESIAN_POINT('Ctrl Pts',(62.0137778853462,-8.25035081906717,30.9041036111461));
#24108=CARTESIAN_POINT('Ctrl Pts',(62.0090864889818,-8.30112520359226,30.8953235179838));
#24109=CARTESIAN_POINT('Origin',(64.,8.48528137423857,13.));
#24110=CARTESIAN_POINT('',(62.,8.48528137423857,30.854497241083));
#24111=CARTESIAN_POINT('',(62.,8.48528137423857,-30.854497241083));
#24112=CARTESIAN_POINT('',(62.,8.48528137423857,13.));
#24113=CARTESIAN_POINT('Ctrl Pts',(62.,8.48528137423857,-30.854497241083));
#24114=CARTESIAN_POINT('Ctrl Pts',(62.,8.42347251099396,-30.8714952686948));
#24115=CARTESIAN_POINT('Ctrl Pts',(62.0029020528202,8.36152602610337,-30.8853188733362));
#24116=CARTESIAN_POINT('Ctrl Pts',(62.0085237302078,8.30083011548887,-30.8958051086952));
#24117=CARTESIAN_POINT('',(63.3333333333334,6.59966329107444,31.7128621774316));
#24118=CARTESIAN_POINT('',(63.3333333333333,6.59966329107444,13.));
#24119=CARTESIAN_POINT('',(62.0088203985241,8.30104700095525,30.8955604966231));
#24120=CARTESIAN_POINT('Ctrl Pts',(63.3333333333334,6.59966329107444,31.7128621774316));
#24121=CARTESIAN_POINT('Ctrl Pts',(63.3315791447087,6.60028349041044,31.7119917027092));
#24122=CARTESIAN_POINT('Ctrl Pts',(63.3298258043253,6.60090614371271,31.7111212674742));
#24123=CARTESIAN_POINT('Ctrl Pts',(63.0820808102159,6.68927586421289,31.5880758676829));
#24124=CARTESIAN_POINT('Ctrl Pts',(62.8535438668757,6.82510864451255,31.46712247015));
#24125=CARTESIAN_POINT('Ctrl Pts',(62.4713648466326,7.17154726287157,31.2499029440192));
#24126=CARTESIAN_POINT('Ctrl Pts',(62.3159333486232,7.37581872562244,31.1536217805848));
#24127=CARTESIAN_POINT('Ctrl Pts',(62.0981396750928,7.82229843047092,30.9982213735624));
#24128=CARTESIAN_POINT('Ctrl Pts',(62.0311590674915,8.05644177565425,30.9380272884007));
#24129=CARTESIAN_POINT('Ctrl Pts',(62.0085237302653,8.30083011486769,30.8958051088025));
#24130=CARTESIAN_POINT('Ctrl Pts',(62.0085237301807,8.30083011578128,30.8958051086446));
#24131=CARTESIAN_POINT('Ctrl Pts',(62.0029032474376,8.36151312820127,30.885321101655));
#24132=CARTESIAN_POINT('Ctrl Pts',(62.,8.42346268655744,30.8714979705087));
#24133=CARTESIAN_POINT('Ctrl Pts',(62.,8.48528137423857,30.854497241083));
#24134=CARTESIAN_POINT('Ctrl Pts',(63.3333333333334,6.59966329107444,31.7128621774316));
#24135=CARTESIAN_POINT('Ctrl Pts',(62.1773896945574,7.00835108389839,33.1107619749047));
#24136=CARTESIAN_POINT('Ctrl Pts',(59.8510643212503,7.17136627556463,36.1604788683916));
#24137=CARTESIAN_POINT('Ctrl Pts',(57.1837550511065,6.08049991760512,40.0089963598732));
#24138=CARTESIAN_POINT('Ctrl Pts',(55.3668248198271,4.31461669518687,42.7323293863949));
#24139=CARTESIAN_POINT('Ctrl Pts',(54.4251147577635,2.64876740625127,44.1726835846802));
#24140=CARTESIAN_POINT('Ctrl Pts',(53.9842189222391,0.833747439766708,44.852770613662));
#24141=CARTESIAN_POINT('Ctrl Pts',(53.985357986249,-0.833764372921021,44.8510072059771));
#24142=CARTESIAN_POINT('Ctrl Pts',(54.3610359933426,-2.38837584180055,44.2714261991957));
#24143=CARTESIAN_POINT('Ctrl Pts',(55.0050244523723,-3.70114923515179,43.2855805513825));
#24144=CARTESIAN_POINT('Ctrl Pts',(55.8180315346338,-4.7647811160322,42.0547184493501));
#24145=CARTESIAN_POINT('Ctrl Pts',(57.3603596238608,-6.15480540711906,39.7540563319785));
#24146=CARTESIAN_POINT('Ctrl Pts',(59.8534489927889,-7.16888802237617,36.1571505333425));
#24147=CARTESIAN_POINT('Ctrl Pts',(62.177413277237,-7.00834274616208,33.1107334560203));
#24148=CARTESIAN_POINT('Ctrl Pts',(63.3333333333333,-6.59966329107444,31.7128621774316));
#24149=CARTESIAN_POINT('Ctrl Pts',(63.1962492273341,6.6481298415469,31.5488996087769));
#24150=CARTESIAN_POINT('Ctrl Pts',(62.0093421297043,7.04072991080625,32.9391773083993));
#24151=CARTESIAN_POINT('Ctrl Pts',(59.6306254735857,7.14629729109621,35.9670702941392));
#24152=CARTESIAN_POINT('Ctrl Pts',(56.9648615533032,5.94454544765156,39.7623544055489));
#24153=CARTESIAN_POINT('Ctrl Pts',(55.2199565629048,4.1186832182827,42.4090274642781));
#24154=CARTESIAN_POINT('Ctrl Pts',(54.3627119956756,2.46990066692426,43.7769112833253));
#24155=CARTESIAN_POINT('Ctrl Pts',(53.9868660380235,0.765082134508059,44.4022644152194));
#24156=CARTESIAN_POINT('Ctrl Pts',(53.9874577061127,-0.764888305104543,
44.40097010027));
#24157=CARTESIAN_POINT('Ctrl Pts',(54.308342330058,-2.22529296405365,43.86757204928));
#24158=CARTESIAN_POINT('Ctrl Pts',(54.8892188306448,-3.5093071402967,42.9356756235718));
#24159=CARTESIAN_POINT('Ctrl Pts',(55.6523321195903,-4.58361797221118,41.7510674504422));
#24160=CARTESIAN_POINT('Ctrl Pts',(57.1409463863557,-6.02588925105485,39.5112017421951));
#24161=CARTESIAN_POINT('Ctrl Pts',(59.6331015208575,-7.14454194899524,35.9635238647728));
#24162=CARTESIAN_POINT('Ctrl Pts',(62.0093663440767,-7.04072190127939,32.9391489450152));
#24163=CARTESIAN_POINT('Ctrl Pts',(63.1962492273341,-6.64812984154691,31.5488996087769));
#24164=CARTESIAN_POINT('Ctrl Pts',(62.9463311105499,6.81360008562125,31.2209941996293));
#24165=CARTESIAN_POINT('Ctrl Pts',(61.6902590726639,7.19193133539315,32.5959957954705));
#24166=CARTESIAN_POINT('Ctrl Pts',(59.1806910892167,7.22376058361478,35.5805693674503));
#24167=CARTESIAN_POINT('Ctrl Pts',(56.4330414247942,5.8407858655779,39.2697861596156));
#24168=CARTESIAN_POINT('Ctrl Pts',(54.7292159564143,3.88448268514588,41.7632982027126));
#24169=CARTESIAN_POINT('Ctrl Pts',(53.9652037659389,2.22577079086734,42.9859075220035));
#24170=CARTESIAN_POINT('Ctrl Pts',(53.6754715503903,0.666318585301244,43.5014342636392));
#24171=CARTESIAN_POINT('Ctrl Pts',(53.6751795362821,-0.665698958814348,
43.501067912247));
#24172=CARTESIAN_POINT('Ctrl Pts',(53.9236778818116,-2.0018479285686,43.0602414260277));
#24173=CARTESIAN_POINT('Ctrl Pts',(54.4317973968295,-3.26780308655164,42.2363800092985));
#24174=CARTESIAN_POINT('Ctrl Pts',(55.1499982747057,-4.38195964414384,41.1445144943703));
#24175=CARTESIAN_POINT('Ctrl Pts',(56.6140690268316,-5.93366160544652,39.0263796051091));
#24176=CARTESIAN_POINT('Ctrl Pts',(59.1836503932084,-7.22318373229117,35.576683205603));
#24177=CARTESIAN_POINT('Ctrl Pts',(61.6902846980866,-7.19192361696785,32.5959677437378));
#24178=CARTESIAN_POINT('Ctrl Pts',(62.9463311105498,-6.81360008562125,31.2209941996293));
#24179=CARTESIAN_POINT('Ctrl Pts',(62.7061595886978,7.20521258113835,30.8184466564059));
#24180=CARTESIAN_POINT('Ctrl Pts',(61.3525918084502,7.61031511383114,32.1841418341021));
#24181=CARTESIAN_POINT('Ctrl Pts',(58.639719444944,7.65453953624728,35.1410478713317));
#24182=CARTESIAN_POINT('Ctrl Pts',(55.6374343951349,6.19012486821752,38.7683214990875));
#24183=CARTESIAN_POINT('Ctrl Pts',(53.7520469534746,4.10519226863261,41.1835161043104));
#24184=CARTESIAN_POINT('Ctrl Pts',(52.8964738416428,2.33969535740793,42.3385222833608));
#24185=CARTESIAN_POINT('Ctrl Pts',(52.5689543596521,0.696894842639347,42.8062051339743));
#24186=CARTESIAN_POINT('Ctrl Pts',(52.5686719868954,-0.69616267180925,42.8062135338103));
#24187=CARTESIAN_POINT('Ctrl Pts',(52.8494705009145,-2.10371014619857,42.405795394335));
#24188=CARTESIAN_POINT('Ctrl Pts',(53.4191785279361,-3.44852229436623,41.6315854149983));
#24189=CARTESIAN_POINT('Ctrl Pts',(54.2179795314303,-4.6354735302374,40.5847140055125));
#24190=CARTESIAN_POINT('Ctrl Pts',(55.8351784344025,-6.28842573724461,38.5292245334429));
#24191=CARTESIAN_POINT('Ctrl Pts',(58.6430771173405,-7.65402260661205,35.1370333846699));
#24192=CARTESIAN_POINT('Ctrl Pts',(61.3526194229065,-7.61030684923857,32.1841139722319));
#24193=CARTESIAN_POINT('Ctrl Pts',(62.7061595886978,-7.20521258113835,30.8184466564059));
#24194=CARTESIAN_POINT('Ctrl Pts',(62.5904039193512,7.6583127936691,30.5250624561551));
#24195=CARTESIAN_POINT('Ctrl Pts',(61.1584933846713,8.11585881641404,31.8989848492516));
#24196=CARTESIAN_POINT('Ctrl Pts',(58.2792017179309,8.24146500383239,34.8758878324567));
#24197=CARTESIAN_POINT('Ctrl Pts',(55.0264864356743,6.82106261533207,38.5566816547643));
#24198=CARTESIAN_POINT('Ctrl Pts',(52.8924820285019,4.67292890435344,41.0602180277437));
#24199=CARTESIAN_POINT('Ctrl Pts',(51.8520940544338,2.76163585714774,42.3048969763665));
#24200=CARTESIAN_POINT('Ctrl Pts',(51.4059275777634,0.845595187901781,42.8430538858222));
#24201=CARTESIAN_POINT('Ctrl Pts',(51.4064422995083,-0.845159328481016,
42.8424354934688));
#24202=CARTESIAN_POINT('Ctrl Pts',(51.7875642574907,-2.48653462782744,42.3826354495856));
#24203=CARTESIAN_POINT('Ctrl Pts',(52.4904256291742,-3.96523549111311,41.5411529134917));
#24204=CARTESIAN_POINT('Ctrl Pts',(53.4212386216903,-5.21989656328882,40.4387210123535));
#24205=CARTESIAN_POINT('Ctrl Pts',(55.2412605277983,-6.91695086253193,38.3135879661086));
#24206=CARTESIAN_POINT('Ctrl Pts',(58.2825427953835,-8.23988638622876,34.872150343801));
#24207=CARTESIAN_POINT('Ctrl Pts',(61.1585225974167,-8.11584948190943,31.898956819536));
#24208=CARTESIAN_POINT('Ctrl Pts',(62.5904039193511,-7.6583127936691,30.5250624561552));
#24209=CARTESIAN_POINT('Ctrl Pts',(62.5777174765496,7.9634392868377,30.3968807187894));
#24210=CARTESIAN_POINT('Ctrl Pts',(61.1076965731432,8.46164972651616,31.7860405531774));
#24211=CARTESIAN_POINT('Ctrl Pts',(58.1492105273372,8.65876024618515,34.8022481083434));
#24212=CARTESIAN_POINT('Ctrl Pts',(54.7703733975909,7.30102209714431,38.5745952960703));
#24213=CARTESIAN_POINT('Ctrl Pts',(52.4937350175267,5.13051425931518,41.2071640355381));
#24214=CARTESIAN_POINT('Ctrl Pts',(51.3344612102292,3.11541106986722,42.5714726656167));
#24215=CARTESIAN_POINT('Ctrl Pts',(50.8048762661169,0.972902268736063,43.1985090979019));
#24216=CARTESIAN_POINT('Ctrl Pts',(50.8060383404805,-0.972769282655253,
43.1971473210877));
#24217=CARTESIAN_POINT('Ctrl Pts',(51.2576003506582,-2.80797998191018,42.6623597404875));
#24218=CARTESIAN_POINT('Ctrl Pts',(52.0476061174834,-4.38726349542764,41.7321453947841));
#24219=CARTESIAN_POINT('Ctrl Pts',(53.0587432961293,-5.68374075190955,40.5526413291701));
#24220=CARTESIAN_POINT('Ctrl Pts',(54.9939048068932,-7.39328817802591,38.3250004905781));
#24221=CARTESIAN_POINT('Ctrl Pts',(58.1523706727149,-8.65618956969658,34.7988022375372));
#24222=CARTESIAN_POINT('Ctrl Pts',(61.1077265633873,-8.46163956240716,31.7860122125991));
#24223=CARTESIAN_POINT('Ctrl Pts',(62.5777174765495,-7.9634392868377,30.3968807187894));
#24224=CARTESIAN_POINT('Ctrl Pts',(62.5857864376269,8.11974451941452,30.3467059609741));
#24225=CARTESIAN_POINT('Ctrl Pts',(61.0995731877722,8.63911281829803,31.7462345485699));
#24226=CARTESIAN_POINT('Ctrl Pts',(58.1085834220916,8.87357929861398,34.7889401279806));
#24227=CARTESIAN_POINT('Ctrl Pts',(54.6791857890496,7.54851825740161,38.6195934717837));
#24228=CARTESIAN_POINT('Ctrl Pts',(52.3431326345475,5.36613894866642,41.3291233333569));
#24229=CARTESIAN_POINT('Ctrl Pts',(51.1323625547514,3.29730168453684,42.7619221061187));
#24230=CARTESIAN_POINT('Ctrl Pts',(50.5654964805058,1.03828559051394,43.4384291646527));
#24231=CARTESIAN_POINT('Ctrl Pts',(50.5669609913757,-1.03830665890786,43.4366729518529));
#24232=CARTESIAN_POINT('Ctrl Pts',(51.0499755719245,-2.97319690488059,42.8601506219393));
#24233=CARTESIAN_POINT('Ctrl Pts',(51.8779607335342,-4.60442848107814,41.8794658901552));
#24234=CARTESIAN_POINT('Ctrl Pts',(52.9232555535846,-5.92265909195242,40.6549664913959));
#24235=CARTESIAN_POINT('Ctrl Pts',(54.9062488111622,-7.63883014775581,38.3658488848707));
#24236=CARTESIAN_POINT('Ctrl Pts',(58.1116494283555,-8.87050844544732,34.7856031628019));
#24237=CARTESIAN_POINT('Ctrl Pts',(61.0996035083602,-8.63910222254255,31.7462059964563));
#24238=CARTESIAN_POINT('Ctrl Pts',(62.5857864376269,-8.11974451941452,30.3467059609741));
#24239=CARTESIAN_POINT('',(62.000165884661,-8.3032680262804,30.9039893606587));
#24240=CARTESIAN_POINT('',(62.0001575703546,8.3032754367448,30.9040190526451));
#24241=CARTESIAN_POINT('Ctrl Pts',(62.0000893809181,-8.30322423863785,30.904080390366));
#24242=CARTESIAN_POINT('Ctrl Pts',(61.6561655749137,-8.39875971217444,31.2347093086726));
#24243=CARTESIAN_POINT('Ctrl Pts',(61.312246656489,-8.47352712664702,31.570965086887));
#24244=CARTESIAN_POINT('Ctrl Pts',(60.9692904429481,-8.52842461676202,31.9113599823671));
#24245=CARTESIAN_POINT('Ctrl Pts',(60.6092687475215,-8.58605380289575,32.2686929086903));
#24246=CARTESIAN_POINT('Ctrl Pts',(60.2503082421953,-8.62178639813802,32.6305870777806));
#24247=CARTESIAN_POINT('Ctrl Pts',(59.8935507198074,-8.63669078438552,32.9952825246954));
#24248=CARTESIAN_POINT('Ctrl Pts',(59.5460504659188,-8.6512084264254,33.3505147270794));
#24249=CARTESIAN_POINT('Ctrl Pts',(59.200640836074,-8.64596508009651,33.7084043749006));
#24250=CARTESIAN_POINT('Ctrl Pts',(58.8584017653847,-8.62197236638857,34.0672926119468));
#24251=CARTESIAN_POINT('Ctrl Pts',(58.6281835464303,-8.6058328887813,34.3087104330332));
#24252=CARTESIAN_POINT('Ctrl Pts',(58.3992449606898,-8.5811865819245,34.5507455964031));
#24253=CARTESIAN_POINT('Ctrl Pts',(58.1718343339284,-8.5483883566638,34.7929625798458));
#24254=CARTESIAN_POINT('Ctrl Pts',(57.7947286563834,-8.49400041035123,35.1946210289467));
#24255=CARTESIAN_POINT('Ctrl Pts',(57.421826114243,-8.41719678346568,35.5967774882034));
#24256=CARTESIAN_POINT('Ctrl Pts',(57.0544150878352,-8.31710533598519,35.9971993560921));
#24257=CARTESIAN_POINT('Ctrl Pts',(56.7092101840014,-8.22306336114325,36.3734199441049));
#24258=CARTESIAN_POINT('Ctrl Pts',(56.368852907092,-8.10846458855582,36.7481092284094));
#24259=CARTESIAN_POINT('Ctrl Pts',(56.0343874284652,-7.97256756446671,37.1194477581821));
#24260=CARTESIAN_POINT('Ctrl Pts',(55.7387207793211,-7.85243493401995,37.4477100925992));
#24261=CARTESIAN_POINT('Ctrl Pts',(55.4476581679515,-7.71565946307753,37.7733539993108));
#24262=CARTESIAN_POINT('Ctrl Pts',(55.1619029604268,-7.56170256232362,38.0951486520963));
#24263=CARTESIAN_POINT('Ctrl Pts',(55.0596996615354,-7.50663828797344,38.2102418305029));
#24264=CARTESIAN_POINT('Ctrl Pts',(54.9581751145601,-7.44937583169452,38.3248428739989));
#24265=CARTESIAN_POINT('Ctrl Pts',(54.857360866142,-7.38988930267797,38.4388964431299));
#24266=CARTESIAN_POINT('Ctrl Pts',(54.6095274878066,-7.24365255853758,38.7192762683279));
#24267=CARTESIAN_POINT('Ctrl Pts',(54.3664530066397,-7.08381787166391,38.9959034963516));
#24268=CARTESIAN_POINT('Ctrl Pts',(54.1286075746492,-6.9100316967836,39.2679453077468));
#24269=CARTESIAN_POINT('Ctrl Pts',(53.8559340081726,-6.71079769967733,39.579822690983));
#24270=CARTESIAN_POINT('Ctrl Pts',(53.5901332063915,-6.4932284863201,39.8856731212024));
#24271=CARTESIAN_POINT('Ctrl Pts',(53.3336133764994,-6.25552348746623,40.1823161614254));
#24272=CARTESIAN_POINT('Ctrl Pts',(53.2023314977896,-6.13387067473281,40.3341323217708));
#24273=CARTESIAN_POINT('Ctrl Pts',(53.073480450123,-6.00694321737372,40.4835370465735));
#24274=CARTESIAN_POINT('Ctrl Pts',(52.9473834727163,-5.87449429652602,40.6301042204462));
#24275=CARTESIAN_POINT('Ctrl Pts',(52.8117095535923,-5.73198601008858,40.787803027374));
#24276=CARTESIAN_POINT('Ctrl Pts',(52.6792238533422,-5.58308587547121,40.9422169831774));
#24277=CARTESIAN_POINT('Ctrl Pts',(52.5504935599745,-5.42758583527421,41.0926023952026));
#24278=CARTESIAN_POINT('Ctrl Pts',(52.3454270557672,-5.17987530177754,41.3321653599177));
#24279=CARTESIAN_POINT('Ctrl Pts',(52.1499225997406,-4.91535186897423,41.561480678128));
#24280=CARTESIAN_POINT('Ctrl Pts',(51.9663979586597,-4.63330475841997,41.7773970455567));
#24281=CARTESIAN_POINT('Ctrl Pts',(51.9489051159833,-4.60642114375545,41.7979773394314));
#24282=CARTESIAN_POINT('Ctrl Pts',(51.9315210899143,-4.57937834572491,41.8184359269166));
#24283=CARTESIAN_POINT('Ctrl Pts',(51.9142479594617,-4.55217576216835,41.8387700961554));
#24284=CARTESIAN_POINT('Ctrl Pts',(51.7536961254005,-4.29933076147783,42.0277739466369));
#24285=CARTESIAN_POINT('Ctrl Pts',(51.6027273490625,-4.03268011577195,42.2060260038393));
#24286=CARTESIAN_POINT('Ctrl Pts',(51.464240637923,-3.75251435206581,42.36988034755));
#24287=CARTESIAN_POINT('Ctrl Pts',(51.3334041833375,-3.4878254521854,42.5246830807737));
#24288=CARTESIAN_POINT('Ctrl Pts',(51.2137091021908,-3.21107414891051,42.6666345143635));
#24289=CARTESIAN_POINT('Ctrl Pts',(51.1075727371426,-2.92250941342542,42.7926932040937));
#24290=CARTESIAN_POINT('Ctrl Pts',(51.0958316745257,-2.89058768116312,42.806638122679));
#24291=CARTESIAN_POINT('Ctrl Pts',(51.0842565032326,-2.85852138158929,42.8203885943635));
#24292=CARTESIAN_POINT('Ctrl Pts',(51.0728507020669,-2.82631478942691,42.8339402661012));
#24293=CARTESIAN_POINT('Ctrl Pts',(50.9905591164766,-2.59394781257042,42.9317140689659));
#24294=CARTESIAN_POINT('Ctrl Pts',(50.9171137635618,-2.35422681405925,43.019113509796));
#24295=CARTESIAN_POINT('Ctrl Pts',(50.8538042492007,-2.10863256818959,43.0945234256458));
#24296=CARTESIAN_POINT('Ctrl Pts',(50.794402771643,-1.87819862423098,43.1652783582842));
#24297=CARTESIAN_POINT('Ctrl Pts',(50.7439241014323,-1.6425934332917,43.2254786846976));
#24298=CARTESIAN_POINT('Ctrl Pts',(50.7034615123714,-1.40302481611627,43.2737571692822));
#24299=CARTESIAN_POINT('Ctrl Pts',(50.691004801656,-1.32927182526984,43.2886200618999));
#24300=CARTESIAN_POINT('Ctrl Pts',(50.6794976055421,-1.25514312052498,43.3023527755394));
#24301=CARTESIAN_POINT('Ctrl Pts',(50.6689724743387,-1.18067377945559,43.3149146392693));
#24302=CARTESIAN_POINT('Ctrl Pts',(50.661175987002,-1.12551064054602,43.3242198355278));
#24303=CARTESIAN_POINT('Ctrl Pts',(50.6539207978311,-1.07017769902012,43.3328796750757));
#24304=CARTESIAN_POINT('Ctrl Pts',(50.6472193363222,-1.01468965833302,43.3408785990006));
#24305=CARTESIAN_POINT('Ctrl Pts',(50.616356722979,-0.759147498968588,43.3777164881572));
#24306=CARTESIAN_POINT('Ctrl Pts',(50.5972357485005,-0.500317544405125,
43.4005398504856));
#24307=CARTESIAN_POINT('Ctrl Pts',(50.5898714711672,-0.240738864968742,
43.4093313537544));
#24308=CARTESIAN_POINT('Ctrl Pts',(50.5875961987457,-0.160539249469542,
43.4120475829275));
#24309=CARTESIAN_POINT('Ctrl Pts',(50.586443408801,-0.0802680232746275,
43.413424106223));
#24310=CARTESIAN_POINT('Ctrl Pts',(50.5864141549312,2.20702370434811E-7,
43.413459684969));
#24311=CARTESIAN_POINT('Ctrl Pts',(50.5863344035338,0.218826128786446,43.4135566791352));
#24312=CARTESIAN_POINT('Ctrl Pts',(50.5946901354538,0.437687451886798,43.4036025250393));
#24313=CARTESIAN_POINT('Ctrl Pts',(50.6114484592242,0.65505550810239,43.3836221739438));
#24314=CARTESIAN_POINT('Ctrl Pts',(50.6207357926489,0.775519203732342,43.3725492178948));
#24315=CARTESIAN_POINT('Ctrl Pts',(50.6326040296411,0.895525157135156,43.3583966672893));
#24316=CARTESIAN_POINT('Ctrl Pts',(50.6470500171268,1.0148189366432,43.3411658012909));
#24317=CARTESIAN_POINT('Ctrl Pts',(50.6472729914877,1.01666024062296,43.3408998422252));
#24318=CARTESIAN_POINT('Ctrl Pts',(50.6474965800171,1.01850137500363,43.3406331497258));
#24319=CARTESIAN_POINT('Ctrl Pts',(50.647720782167,1.02034233925431,43.3403657244623));
#24320=CARTESIAN_POINT('Ctrl Pts',(50.6735956285347,1.23280536498562,43.3095025609724));
#24321=CARTESIAN_POINT('Ctrl Pts',(50.7075375601688,1.44282541763031,43.2689898459162));
#24322=CARTESIAN_POINT('Ctrl Pts',(50.7488174201003,1.6495499391546,43.2197515368914));
#24323=CARTESIAN_POINT('Ctrl Pts',(50.7926945580034,1.86928131309695,43.1674152140748));
#24324=CARTESIAN_POINT('Ctrl Pts',(50.8448629741679,2.08528923107664,43.1052195558173));
#24325=CARTESIAN_POINT('Ctrl Pts',(50.9044498982716,2.29649084950969,43.0342719592216));
#24326=CARTESIAN_POINT('Ctrl Pts',(50.9301517198461,2.38758912979296,43.0036699018697));
#24327=CARTESIAN_POINT('Ctrl Pts',(50.9572336936552,2.4777925102904,42.9714396437231));
#24328=CARTESIAN_POINT('Ctrl Pts',(50.985625379792,2.56701126801593,42.9376706686577));
#24329=CARTESIAN_POINT('Ctrl Pts',(51.0239835929914,2.6875490942565,42.8920475401528));
#24330=CARTESIAN_POINT('Ctrl Pts',(51.0647374564426,2.80638398422016,42.8436050676676));
#24331=CARTESIAN_POINT('Ctrl Pts',(51.1076949778189,2.92327958149374,42.7925812475125));
#24332=CARTESIAN_POINT('Ctrl Pts',(51.1859073117987,3.13611023842693,42.6996826831855));
#24333=CARTESIAN_POINT('Ctrl Pts',(51.2714261489779,3.34250990315628,42.5982253582903));
#24334=CARTESIAN_POINT('Ctrl Pts',(51.3633720424189,3.54236397232683,42.4893210803475));
#24335=CARTESIAN_POINT('Ctrl Pts',(51.4601407745289,3.75270098855345,42.3747044454606));
#24336=CARTESIAN_POINT('Ctrl Pts',(51.5640280213028,3.95578770363038,42.2518397579902));
#24337=CARTESIAN_POINT('Ctrl Pts',(51.6739780854953,4.1515305695143,42.1220580223104));
#24338=CARTESIAN_POINT('Ctrl Pts',(51.7933202450361,4.36399407738818,41.9811901408886));
#24339=CARTESIAN_POINT('Ctrl Pts',(51.919804621899,4.56780518704684,41.832173867876));
#24340=CARTESIAN_POINT('Ctrl Pts',(52.0520547200304,4.76289322778432,41.6767397588155));
#24341=CARTESIAN_POINT('Ctrl Pts',(52.1214830965618,4.86531013439127,41.5951402893094));
#24342=CARTESIAN_POINT('Ctrl Pts',(52.1925001533719,4.9653237612545,41.5117724248637));
#24343=CARTESIAN_POINT('Ctrl Pts',(52.2649051712575,5.06292908031616,41.4268879616273));
#24344=CARTESIAN_POINT('Ctrl Pts',(52.3120967308617,5.12654548932615,41.3715626496079));
#24345=CARTESIAN_POINT('Ctrl Pts',(52.3599068618714,5.18916334778516,41.3155609124478));
#24346=CARTESIAN_POINT('Ctrl Pts',(52.4082860638065,5.25078255038662,41.2589457946924));
#24347=CARTESIAN_POINT('Ctrl Pts',(52.7202424682068,5.64811247970936,40.8938829605977));
#24348=CARTESIAN_POINT('Ctrl Pts',(53.0558615152328,6.00392110101613,40.5033140822927));
#24349=CARTESIAN_POINT('Ctrl Pts',(53.4085173529738,6.32279271823725,40.0959222298945));
#24350=CARTESIAN_POINT('Ctrl Pts',(53.641979521913,6.53388934957749,39.826224197733));
#24351=CARTESIAN_POINT('Ctrl Pts',(53.8829080025842,6.72879759239876,39.5491538062669));
#24352=CARTESIAN_POINT('Ctrl Pts',(54.1293733297254,6.90884566929533,39.2672410660208));
#24353=CARTESIAN_POINT('Ctrl Pts',(54.2994228263867,7.03307038360392,39.0727345196546));
#24354=CARTESIAN_POINT('Ctrl Pts',(54.4721077718443,7.15022117656695,38.875923214831));
#24355=CARTESIAN_POINT('Ctrl Pts',(54.6472464829213,7.26041604117073,38.6771203410467));
#24356=CARTESIAN_POINT('Ctrl Pts',(54.9696401158298,7.46326167426362,38.3111659479952));
#24357=CARTESIAN_POINT('Ctrl Pts',(55.2997861374957,7.6426576925173,37.9390118616385));
#24358=CARTESIAN_POINT('Ctrl Pts',(55.6365936394474,7.79941676002793,37.5625544660927));
#24359=CARTESIAN_POINT('Ctrl Pts',(56.0062120435004,7.97144688411473,37.1494235799654));
#24360=CARTESIAN_POINT('Ctrl Pts',(56.3838529220466,8.11621342061613,36.7311104385792));
#24361=CARTESIAN_POINT('Ctrl Pts',(56.7680476094898,8.23474387868071,36.3101601802102));
#24362=CARTESIAN_POINT('Ctrl Pts',(57.1913088001799,8.36532700346917,35.8464059602747));
#24363=CARTESIAN_POINT('Ctrl Pts',(57.6225246054172,8.46406571536722,35.3794511113515));
#24364=CARTESIAN_POINT('Ctrl Pts',(58.0596999375003,8.53230441069762,34.9127398648411));
#24365=CARTESIAN_POINT('Ctrl Pts',(58.0966419874149,8.53807069507829,34.8733019805439));
#24366=CARTESIAN_POINT('Ctrl Pts',(58.1336265730028,8.54361918421598,34.8338658580828));
#24367=CARTESIAN_POINT('Ctrl Pts',(58.170652480092,8.54895068510073,34.7944335879392));
#24368=CARTESIAN_POINT('Ctrl Pts',(58.5551743043278,8.60431944193314,34.3849211778079));
#24369=CARTESIAN_POINT('Ctrl Pts',(58.9441544561351,8.63628571489729,33.9758224439262));
#24370=CARTESIAN_POINT('Ctrl Pts',(59.336276225615,8.64326314471869,33.5693475219187));
#24371=CARTESIAN_POINT('Ctrl Pts',(59.658536886301,8.64899746328794,33.235290891775));
#24372=CARTESIAN_POINT('Ctrl Pts',(59.9831665395922,8.63812999453601,32.9026794425133));
#24373=CARTESIAN_POINT('Ctrl Pts',(60.3092847224631,8.60972594452936,32.5729022773846));
#24374=CARTESIAN_POINT('Ctrl Pts',(60.6235699359896,8.58235251553876,32.255090845203));
#24375=CARTESIAN_POINT('Ctrl Pts',(60.9392371253881,8.53869186336392,31.9399124481438));
#24376=CARTESIAN_POINT('Ctrl Pts',(61.2554899897929,8.47795384680794,31.6286113065427));
#24377=CARTESIAN_POINT('Ctrl Pts',(61.5034619132754,8.43032954205346,31.3845219984178));
#24378=CARTESIAN_POINT('Ctrl Pts',(61.751793684675,8.37220685580352,31.1428165614412));
#24379=CARTESIAN_POINT('Ctrl Pts',(62.0001005262926,8.30322713190806,30.9040911403702));
#24380=CARTESIAN_POINT('Ctrl Pts',(62.0090216939304,8.30119416254679,30.8953945223182));
#24381=CARTESIAN_POINT('Ctrl Pts',(62.0061846213717,8.30198895980305,30.8981203196454));
#24382=CARTESIAN_POINT('Ctrl Pts',(62.0033475485117,8.30278233098926,30.9008465054417));
#24383=CARTESIAN_POINT('Ctrl Pts',(62.0005104758444,8.30357427665019,30.9035730788998));
#24384=CARTESIAN_POINT('',(54.0004882446407,-5.63129358982506E-5,44.8276698544958));
#24385=CARTESIAN_POINT('Ctrl Pts',(63.3333333333334,6.59966329107444,31.7128621774316));
#24386=CARTESIAN_POINT('Ctrl Pts',(62.1773896945574,7.00835108389839,33.1107619749047));
#24387=CARTESIAN_POINT('Ctrl Pts',(59.8510643212503,7.17136627556463,36.1604788683916));
#24388=CARTESIAN_POINT('Ctrl Pts',(57.1837550511065,6.08049991760512,40.0089963598732));
#24389=CARTESIAN_POINT('Ctrl Pts',(55.3668248198271,4.31461669518687,42.7323293863949));
#24390=CARTESIAN_POINT('Ctrl Pts',(54.4251147577635,2.64876740625127,44.1726835846802));
#24391=CARTESIAN_POINT('Ctrl Pts',(54.0471985724064,1.0930134915766,44.7556237601027));
#24392=CARTESIAN_POINT('Ctrl Pts',(54.0003896413325,0.273205195412317,44.8278246929999));
#24393=CARTESIAN_POINT('Ctrl Pts',(54.0004882446406,-5.63129358982679E-5,
44.8276698544958));
#24394=CARTESIAN_POINT('Ctrl Pts',(54.0004882243341,5.92031391855041E-7,
44.8276698863898));
#24395=CARTESIAN_POINT('Ctrl Pts',(54.0005846376296,-0.273232435743518,
44.8275184265616));
#24396=CARTESIAN_POINT('Ctrl Pts',(54.0479720776823,-1.09287079602173,44.7544086895179));
#24397=CARTESIAN_POINT('Ctrl Pts',(54.3610359933426,-2.38837584180055,44.2714261991957));
#24398=CARTESIAN_POINT('Ctrl Pts',(55.0050244523723,-3.70114923515179,43.2855805513825));
#24399=CARTESIAN_POINT('Ctrl Pts',(55.8180315346338,-4.7647811160322,42.0547184493501));
#24400=CARTESIAN_POINT('Ctrl Pts',(57.3603596238608,-6.15480540711906,39.7540563319785));
#24401=CARTESIAN_POINT('Ctrl Pts',(59.8534489927889,-7.16888802237617,36.1571505333425));
#24402=CARTESIAN_POINT('Ctrl Pts',(62.177413277237,-7.00834274616208,33.1107334560203));
#24403=CARTESIAN_POINT('Ctrl Pts',(63.3333333333333,-6.59966329107444,31.7128621774316));
#24404=CARTESIAN_POINT('Ctrl Pts',(62.0090864865565,-8.30112520427131,30.8953235203139));
#24405=CARTESIAN_POINT('Ctrl Pts',(62.0062500143164,-8.30191935890931,30.8980486593436));
#24406=CARTESIAN_POINT('Ctrl Pts',(62.0034135456646,-8.30271208344451,30.9007741826053));
#24407=CARTESIAN_POINT('Ctrl Pts',(62.0005770810725,-8.3035033784451,30.9035000893158));
#24408=CARTESIAN_POINT('Origin',(62.,0.,0.));
#24409=CARTESIAN_POINT('',(62.,-32.,-3.91886975727153E-15));
#24410=CARTESIAN_POINT('Origin',(62.,0.,0.));
#24411=CARTESIAN_POINT('Origin',(62.,0.,0.));
#24412=CARTESIAN_POINT('Origin',(61.,0.,13.));
#24413=CARTESIAN_POINT('',(54.,-8.57252759403147E-16,-50.));
#24414=CARTESIAN_POINT('Origin',(61.,0.,-50.));
#24415=CARTESIAN_POINT('',(54.,-8.57252759403147E-16,13.));
#24416=CARTESIAN_POINT('',(54.,-8.57252759403147E-16,76.));
#24417=CARTESIAN_POINT('',(54.,-8.57252759403147E-16,13.));
#24418=CARTESIAN_POINT('Origin',(61.,0.,76.));
#24419=CARTESIAN_POINT('Origin',(53.,-25.,-65.));
#24420=CARTESIAN_POINT('',(53.,-33.,-65.));
#24421=CARTESIAN_POINT('Origin',(53.,-25.,-65.));
#24422=CARTESIAN_POINT('',(53.,-31.,-63.));
#24423=CARTESIAN_POINT('Origin',(53.,-31.,-65.));
#24424=CARTESIAN_POINT('Origin',(53.,-25.,-63.));
#24425=CARTESIAN_POINT('Origin',(57.,-31.,-65.));
#24426=CARTESIAN_POINT('',(61.776208734813,-31.,-63.));
#24427=CARTESIAN_POINT('',(60.2237912651869,-31.,-63.));
#24428=CARTESIAN_POINT('Ctrl Pts',(61.7762087348131,-31.,-63.));
#24429=CARTESIAN_POINT('Ctrl Pts',(61.7599416865592,-31.0010478526925,-63.));
#24430=CARTESIAN_POINT('Ctrl Pts',(61.7436725835362,-31.0020628978659,-63.0000008227015));
#24431=CARTESIAN_POINT('Ctrl Pts',(61.4851779611869,-31.0176669941819,-63.0000245808219));
#24432=CARTESIAN_POINT('Ctrl Pts',(61.2426971526137,-31.0249999999999,-63.000156256104));
#24433=CARTESIAN_POINT('Ctrl Pts',(60.7573028473861,-31.0249999999999,-63.000156256104));
#24434=CARTESIAN_POINT('Ctrl Pts',(60.5148220388123,-31.0176669941818,-63.0000245808219));
#24435=CARTESIAN_POINT('Ctrl Pts',(60.256327416464,-31.002062897866,-63.0000008227015));
#24436=CARTESIAN_POINT('Ctrl Pts',(60.2400583134407,-31.0010478526925,-63.));
#24437=CARTESIAN_POINT('Ctrl Pts',(60.2237912651869,-31.,-63.));
#24438=CARTESIAN_POINT('',(57.,-31.,-63.));
#24439=CARTESIAN_POINT('',(69.,-33.,-65.));
#24440=CARTESIAN_POINT('',(57.,-33.,-65.));
#24441=CARTESIAN_POINT('',(69.,-31.,-63.));
#24442=CARTESIAN_POINT('Origin',(69.,-31.,-65.));
#24443=CARTESIAN_POINT('',(57.,-31.,-63.));
#24444=CARTESIAN_POINT('Origin',(69.,-25.,-65.));
#24445=CARTESIAN_POINT('',(77.,-25.,-65.));
#24446=CARTESIAN_POINT('',(75.,-25.,-63.));
#24447=CARTESIAN_POINT('Origin',(75.,-25.,-65.));
#24448=CARTESIAN_POINT('Origin',(69.,-25.,-63.));
#24449=CARTESIAN_POINT('Origin',(69.,-25.,-65.));
#24450=CARTESIAN_POINT('Origin',(75.,-7.,-65.));
#24451=CARTESIAN_POINT('',(77.,-14.,-65.));
#24452=CARTESIAN_POINT('',(75.,-19.2915026221292,-63.));
#24453=CARTESIAN_POINT('Ctrl Pts',(75.,-19.2915026221292,-63.));
#24454=CARTESIAN_POINT('Ctrl Pts',(75.6598443730912,-18.5433094298986,-63.));
#24455=CARTESIAN_POINT('Ctrl Pts',(76.1700160324087,-17.6794947918718,-63.2991643782353));
#24456=CARTESIAN_POINT('Ctrl Pts',(76.8431824332822,-15.8525818385792,-64.0701256324549));
#24457=CARTESIAN_POINT('Ctrl Pts',(77.,-14.8922724470027,-64.5538637764986));
#24458=CARTESIAN_POINT('Ctrl Pts',(77.,-14.,-65.));
#24459=CARTESIAN_POINT('',(75.,-7.,-63.));
#24460=CARTESIAN_POINT('',(77.,-7.,-65.));
#24461=CARTESIAN_POINT('Origin',(53.,-33.,-77.));
#24462=CARTESIAN_POINT('',(53.,-33.,-75.));
#24463=CARTESIAN_POINT('',(53.,-33.,-77.));
#24464=CARTESIAN_POINT('',(69.,-33.,-75.));
#24465=CARTESIAN_POINT('',(57.,-33.,-75.));
#24466=CARTESIAN_POINT('',(69.,-33.,-77.));
#24467=CARTESIAN_POINT('Origin',(53.,-25.,-77.));
#24468=CARTESIAN_POINT('',(45.,-25.,-75.));
#24469=CARTESIAN_POINT('',(45.,-25.,-77.));
#24470=CARTESIAN_POINT('Origin',(53.,-25.,-75.));
#24471=CARTESIAN_POINT('Origin',(61.,0.,-63.));
#24472=CARTESIAN_POINT('Origin',(61.,-25.,-63.));
#24473=CARTESIAN_POINT('Origin',(53.,-14.,-63.));
#24474=CARTESIAN_POINT('Origin',(61.,-25.,-65.));
#24475=CARTESIAN_POINT('Origin',(61.,-25.,-63.));
#24476=CARTESIAN_POINT('Origin',(69.,25.,-75.));
#24477=CARTESIAN_POINT('',(77.,25.,-75.));
#24478=CARTESIAN_POINT('Origin',(75.,25.,-75.));
#24479=CARTESIAN_POINT('',(69.,33.,-75.));
#24480=CARTESIAN_POINT('Origin',(69.,31.,-75.));
#24481=CARTESIAN_POINT('Origin',(69.,25.,-75.));
#24482=CARTESIAN_POINT('Origin',(65.,31.,-75.));
#24483=CARTESIAN_POINT('',(53.,33.,-75.));
#24484=CARTESIAN_POINT('Origin',(53.,31.,-75.));
#24485=CARTESIAN_POINT('',(65.,33.,-75.));
#24486=CARTESIAN_POINT('Origin',(53.,25.,-75.));
#24487=CARTESIAN_POINT('',(45.,25.,-75.));
#24488=CARTESIAN_POINT('Origin',(47.,25.,-75.));
#24489=CARTESIAN_POINT('Origin',(53.,25.,-75.));
#24490=CARTESIAN_POINT('Origin',(47.,7.,-75.));
#24491=CARTESIAN_POINT('Origin',(47.,-25.,-75.));
#24492=CARTESIAN_POINT('',(45.,7.,-75.));
#24493=CARTESIAN_POINT('Origin',(53.,-25.,-75.));
#24494=CARTESIAN_POINT('Origin',(53.,-31.,-75.));
#24495=CARTESIAN_POINT('Origin',(57.,-31.,-75.));
#24496=CARTESIAN_POINT('Origin',(69.,-31.,-75.));
#24497=CARTESIAN_POINT('Origin',(69.,-25.,-75.));
#24498=CARTESIAN_POINT('',(77.,-25.,-75.));
#24499=CARTESIAN_POINT('Origin',(75.,-25.,-75.));
#24500=CARTESIAN_POINT('Origin',(69.,-25.,-75.));
#24501=CARTESIAN_POINT('Origin',(75.,-7.,-75.));
#24502=CARTESIAN_POINT('',(77.,-7.,-75.));
#24503=CARTESIAN_POINT('Origin',(69.,-25.,-77.));
#24504=CARTESIAN_POINT('',(77.,-25.,-77.));
#24505=CARTESIAN_POINT('Origin',(77.,-14.,-77.));
#24506=CARTESIAN_POINT('',(77.,25.,-65.));
#24507=CARTESIAN_POINT('',(77.,25.,-77.));
#24508=CARTESIAN_POINT('',(77.,14.,-65.));
#24509=CARTESIAN_POINT('',(77.,-7.,-65.));
#24510=CARTESIAN_POINT('',(77.,14.,-77.));
#24511=CARTESIAN_POINT('',(77.,-14.,-77.));
#24512=CARTESIAN_POINT('Origin',(69.,25.,-77.));
#24513=CARTESIAN_POINT('',(69.,33.,-65.));
#24514=CARTESIAN_POINT('',(69.,33.,-77.));
#24515=CARTESIAN_POINT('Origin',(69.,25.,-65.));
#24516=CARTESIAN_POINT('Origin',(75.,-7.,-65.));
#24517=CARTESIAN_POINT('',(75.,25.,-63.));
#24518=CARTESIAN_POINT('Origin',(75.,25.,-65.));
#24519=CARTESIAN_POINT('',(75.,19.2915026221292,-63.));
#24520=CARTESIAN_POINT('',(75.,-7.,-63.));
#24521=CARTESIAN_POINT('Ctrl Pts',(77.,14.,-65.));
#24522=CARTESIAN_POINT('Ctrl Pts',(77.,14.8922724470027,-64.5538637764986));
#24523=CARTESIAN_POINT('Ctrl Pts',(76.8431824332822,15.8525818385793,-64.0701256324549));
#24524=CARTESIAN_POINT('Ctrl Pts',(76.1700160324087,17.6794947918718,-63.2991643782353));
#24525=CARTESIAN_POINT('Ctrl Pts',(75.6598443730912,18.5433094298986,-63.));
#24526=CARTESIAN_POINT('Ctrl Pts',(75.,19.2915026221292,-63.));
#24527=CARTESIAN_POINT('Origin',(69.,25.,-65.));
#24528=CARTESIAN_POINT('',(69.,31.,-63.));
#24529=CARTESIAN_POINT('Origin',(69.,31.,-65.));
#24530=CARTESIAN_POINT('Origin',(69.,25.,-63.));
#24531=CARTESIAN_POINT('Origin',(65.,31.,-65.));
#24532=CARTESIAN_POINT('',(60.2237912651869,31.,-63.));
#24533=CARTESIAN_POINT('',(61.776208734813,31.,-63.));
#24534=CARTESIAN_POINT('Ctrl Pts',(60.2237912651869,31.,-63.));
#24535=CARTESIAN_POINT('Ctrl Pts',(60.2400583134408,31.0010478526925,-63.));
#24536=CARTESIAN_POINT('Ctrl Pts',(60.2563274164638,31.0020628978659,-63.0000008227015));
#24537=CARTESIAN_POINT('Ctrl Pts',(60.5148220388131,31.0176669941819,-63.0000245808219));
#24538=CARTESIAN_POINT('Ctrl Pts',(60.7573028473863,31.0249999999999,-63.000156256104));
#24539=CARTESIAN_POINT('Ctrl Pts',(61.2426971526137,31.0249999999999,-63.000156256104));
#24540=CARTESIAN_POINT('Ctrl Pts',(61.4851779611869,31.0176669941819,-63.0000245808219));
#24541=CARTESIAN_POINT('Ctrl Pts',(61.7436725835362,31.0020628978659,-63.0000008227015));
#24542=CARTESIAN_POINT('Ctrl Pts',(61.7599416865592,31.0010478526925,-63.));
#24543=CARTESIAN_POINT('Ctrl Pts',(61.7762087348131,31.,-63.));
#24544=CARTESIAN_POINT('',(65.,31.,-63.));
#24545=CARTESIAN_POINT('',(53.,33.,-65.));
#24546=CARTESIAN_POINT('',(65.,33.,-65.));
#24547=CARTESIAN_POINT('',(53.,31.,-63.));
#24548=CARTESIAN_POINT('Origin',(53.,31.,-65.));
#24549=CARTESIAN_POINT('',(65.,31.,-63.));
#24550=CARTESIAN_POINT('Origin',(53.,25.,-65.));
#24551=CARTESIAN_POINT('Origin',(53.,25.,-63.));
#24552=CARTESIAN_POINT('Origin',(53.,25.,-65.));
#24553=CARTESIAN_POINT('Origin',(61.,0.,-63.));
#24554=CARTESIAN_POINT('Origin',(53.,14.,-63.));
#24555=CARTESIAN_POINT('Origin',(61.,25.,-63.));
#24556=CARTESIAN_POINT('Origin',(61.,0.,-63.));
#24557=CARTESIAN_POINT('Origin',(61.,25.,-63.));
#24558=CARTESIAN_POINT('Origin',(69.,14.,-63.));
#24559=CARTESIAN_POINT('Origin',(61.,25.,-65.));
#24560=CARTESIAN_POINT('Origin',(80.,2.,-8.));
#24561=CARTESIAN_POINT('Origin',(80.,-1.11022302462516E-15,-8.));
#24562=CARTESIAN_POINT('Origin',(80.,-4.9960036108132E-15,-26.75));
#24563=CARTESIAN_POINT('Origin',(80.,-6.10622663543836E-15,-33.));
#24564=CARTESIAN_POINT('Origin',(80.,5.92820323027551,5.73205080756888));
#24565=CARTESIAN_POINT('Origin',(80.,6.92820323027551,4.));
#24566=CARTESIAN_POINT('Origin',(80.,23.1661795512337,13.375));
#24567=CARTESIAN_POINT('Origin',(80.,28.5788383248865,16.5));
#24568=CARTESIAN_POINT('Origin',(80.,-2.,8.));
#24569=CARTESIAN_POINT('Origin',(80.,2.77555756156289E-16,8.));
#24570=CARTESIAN_POINT('Origin',(80.,1.80411241501588E-15,26.75));
#24571=CARTESIAN_POINT('Origin',(80.,2.22044604925031E-15,33.));
#24572=CARTESIAN_POINT('Origin',(80.,-7.92820323027551,2.26794919243112));
#24573=CARTESIAN_POINT('Origin',(80.,-6.92820323027551,4.));
#24574=CARTESIAN_POINT('Origin',(80.,-23.1661795512337,13.375));
#24575=CARTESIAN_POINT('Origin',(80.,-28.5788383248865,16.5));
#24576=CARTESIAN_POINT('Origin',(80.,-5.92820323027551,-5.73205080756888));
#24577=CARTESIAN_POINT('Origin',(80.,-6.92820323027551,-4.));
#24578=CARTESIAN_POINT('Origin',(80.,-23.1661795512337,-13.375));
#24579=CARTESIAN_POINT('Origin',(80.,-28.5788383248865,-16.5));
#24580=CARTESIAN_POINT('Origin',(80.,7.92820323027551,-2.26794919243113));
#24581=CARTESIAN_POINT('Origin',(80.,6.92820323027551,-4.));
#24582=CARTESIAN_POINT('Origin',(80.,23.1661795512337,-13.375));
#24583=CARTESIAN_POINT('Origin',(80.,28.5788383248865,-16.5));
#24584=CARTESIAN_POINT('Origin',(80.,27.5788383248865,-18.2320508075689));
#24585=CARTESIAN_POINT('Origin',(80.,-29.5788383248865,-14.7679491924311));
#24586=CARTESIAN_POINT('Origin',(80.,-27.5788383248865,18.2320508075689));
#24587=CARTESIAN_POINT('Origin',(80.,2.,33.));
#24588=CARTESIAN_POINT('Origin',(80.,29.5788383248865,14.7679491924311));
#24589=CARTESIAN_POINT('Origin',(80.,-2.00000000000001,-33.));
#24590=CARTESIAN_POINT('Origin',(61.,25.,68.));
#24591=CARTESIAN_POINT('Origin',(61.,-25.,68.));
#24592=CARTESIAN_POINT('Origin',(61.,25.,-63.));
#24593=CARTESIAN_POINT('Origin',(61.,-25.,-63.));
#24594=CARTESIAN_POINT('Origin',(61.,0.,-63.));
#24595=CARTESIAN_POINT('Origin',(69.,-14.,-63.));
#24596=CARTESIAN_POINT('Origin',(38.,-31.,-53.6935750346352));
#24597=CARTESIAN_POINT('',(38.,-31.,-49.1935750346352));
#24598=CARTESIAN_POINT('Origin',(38.,62.,0.));
#24599=CARTESIAN_POINT('',(38.,62.,4.5));
#24600=CARTESIAN_POINT('Origin',(38.,31.,53.6935750346352));
#24601=CARTESIAN_POINT('',(38.,31.,58.1935750346352));
#24602=CARTESIAN_POINT('Origin',(38.,-31.,53.6935750346352));
#24603=CARTESIAN_POINT('',(38.,-31.,58.1935750346352));
#24604=CARTESIAN_POINT('Origin',(38.,-62.,7.59281015471359E-15));
#24605=CARTESIAN_POINT('',(38.,-62.,4.50000000000001));
#24606=CARTESIAN_POINT('Origin',(38.,31.,-53.6935750346352));
#24607=CARTESIAN_POINT('',(38.,31.,-49.1935750346352));
#24608=CARTESIAN_POINT('Origin',(61.,0.,-74.05));
#24609=CARTESIAN_POINT('',(47.95,-1.5981640728873E-15,-71.));
#24610=CARTESIAN_POINT('',(47.95,-1.5981640728873E-15,-74.05));
#24611=CARTESIAN_POINT('Origin',(61.,0.,-71.));
#24612=CARTESIAN_POINT('Origin',(72.,0.,-71.));
#24613=CARTESIAN_POINT('',(50.,-1.34711147906209E-15,-71.));
#24614=CARTESIAN_POINT('Origin',(61.,0.,-71.));
#24615=CARTESIAN_POINT('Origin',(61.,0.,-60.5));
#24616=CARTESIAN_POINT('',(50.,-1.34711147906209E-15,-50.));
#24617=CARTESIAN_POINT('',(50.,-1.34711147906209E-15,-60.5));
#24618=CARTESIAN_POINT('Origin',(61.,0.,-50.));
#24619=CARTESIAN_POINT('Origin',(68.,0.,-50.));
#24620=CARTESIAN_POINT('Origin',(74.05,0.,76.));
#24621=CARTESIAN_POINT('',(47.95,-1.5981640728873E-15,76.));
#24622=CARTESIAN_POINT('Origin',(61.,0.,76.));
#24623=CARTESIAN_POINT('Origin',(61.,0.,79.05));
#24624=CARTESIAN_POINT('',(47.95,-1.5981640728873E-15,79.05));
#24625=CARTESIAN_POINT('Origin',(56.,0.,0.));
#24626=CARTESIAN_POINT('',(56.,-38.,-4.65365783675994E-15));
#24627=CARTESIAN_POINT('Origin',(62.,0.,0.));
#24628=CARTESIAN_POINT('Origin',(62.,0.,0.));
#24629=CARTESIAN_POINT('Origin',(69.,-25.,65.));
#24630=CARTESIAN_POINT('',(69.,-33.,65.));
#24631=CARTESIAN_POINT('Origin',(53.,-33.,65.));
#24632=CARTESIAN_POINT('',(53.,-33.,65.));
#24633=CARTESIAN_POINT('Origin',(53.,-25.,65.));
#24634=CARTESIAN_POINT('',(45.,-25.,65.));
#24635=CARTESIAN_POINT('Origin',(53.,25.,-77.));
#24636=CARTESIAN_POINT('',(45.,25.,-77.));
#24637=CARTESIAN_POINT('',(53.,33.,-77.));
#24638=CARTESIAN_POINT('Origin',(69.,33.,-77.));
#24639=CARTESIAN_POINT('Origin',(53.,14.,-77.));
#24640=CARTESIAN_POINT('Origin',(45.,14.,-77.));
#24641=CARTESIAN_POINT('Origin',(45.,14.,-77.));
#24642=CARTESIAN_POINT('Origin',(53.,-14.,-77.));
#24643=CARTESIAN_POINT('Origin',(53.,-14.,-77.));
#24644=CARTESIAN_POINT('',(53.,-22.,-77.));
#24645=CARTESIAN_POINT('Origin',(69.,14.,-77.));
#24646=CARTESIAN_POINT('Origin',(69.,-14.,-77.));
#24647=CARTESIAN_POINT('Origin',(53.,-22.,-77.));
#24648=CARTESIAN_POINT('',(69.,-22.,-77.));
#24649=CARTESIAN_POINT('Origin',(53.,14.,-77.));
#24650=CARTESIAN_POINT('',(53.,22.,-77.));
#24651=CARTESIAN_POINT('Origin',(69.,22.,-77.));
#24652=CARTESIAN_POINT('',(69.,22.,-77.));
#24653=CARTESIAN_POINT('Origin',(69.,14.,-77.));
#24654=CARTESIAN_POINT('Origin',(69.,-14.,-77.));
#56597=UNCERTAINTY_MEASURE_WITH_UNIT(LENGTH_MEASURE(0.01),#56640,
'DISTANCE_ACCURACY_VALUE',
'Maximum model space distance between geometric entities at asserted c
onnectivities');
#56617=UNCERTAINTY_MEASURE_WITH_UNIT(LENGTH_MEASURE(0.01),#56640,
'DISTANCE_ACCURACY_VALUE',
'Maximum model space distance between geometric entities at asserted c
onnectivities');
#56619=(
GEOMETRIC_REPRESENTATION_CONTEXT(3)
GLOBAL_UNCERTAINTY_ASSIGNED_CONTEXT((#56597))
GLOBAL_UNIT_ASSIGNED_CONTEXT((#56640,#56642,#56643))
REPRESENTATION_CONTEXT('','3D')
);
#56639=(
GEOMETRIC_REPRESENTATION_CONTEXT(3)
GLOBAL_UNCERTAINTY_ASSIGNED_CONTEXT((#56617))
GLOBAL_UNIT_ASSIGNED_CONTEXT((#56640,#56642,#56643))
REPRESENTATION_CONTEXT('','3D')
);
#56640=(
LENGTH_UNIT()
NAMED_UNIT(*)
SI_UNIT(.MILLI.,.METRE.)
);
#56642=(
NAMED_UNIT(*)
PLANE_ANGLE_UNIT()
SI_UNIT($,.RADIAN.)
);
#56643=(
NAMED_UNIT(*)
SI_UNIT($,.STERADIAN.)
SOLID_ANGLE_UNIT()
);
#56645=SHAPE_DEFINITION_REPRESENTATION(#56666,#56745);
#56666=PRODUCT_DEFINITION_SHAPE('',$,#56767);
#56745=SHAPE_REPRESENTATION('',(#17191),#56619);
#56765=PRODUCT_DEFINITION_CONTEXT('part definition',#56830,'design');
#56767=PRODUCT_DEFINITION('2026-10-26-00-02-35-941',
'01_Out_Chamber_ADC12',#56788,#56765);
#56788=PRODUCT_DEFINITION_FORMATION('',$,#56833);
#56830=APPLICATION_CONTEXT(
'Core Data for Automotive Mechanical Design Process');
#56831=PRODUCT_CONTEXT('part definition',#56830,'mechanical');
#56833=PRODUCT('2026-10-26-00-02-35-941','01_Out_Chamber_ADC12',$,(#56831));
#56902=COLOUR_RGB('Sky Blue',0.24,0.69,0.87);
#56903=FILL_AREA_STYLE_COLOUR('',#56902);
#56904=FILL_AREA_STYLE('',(#56903));
#56905=SURFACE_STYLE_FILL_AREA(#56904);
#56906=SURFACE_SIDE_STYLE('',(#56905));
#56907=SURFACE_STYLE_USAGE(.BOTH.,#56906);
#56908=PRESENTATION_STYLE_ASSIGNMENT((#56907));
ENDSEC;
END-ISO-10303-21;
